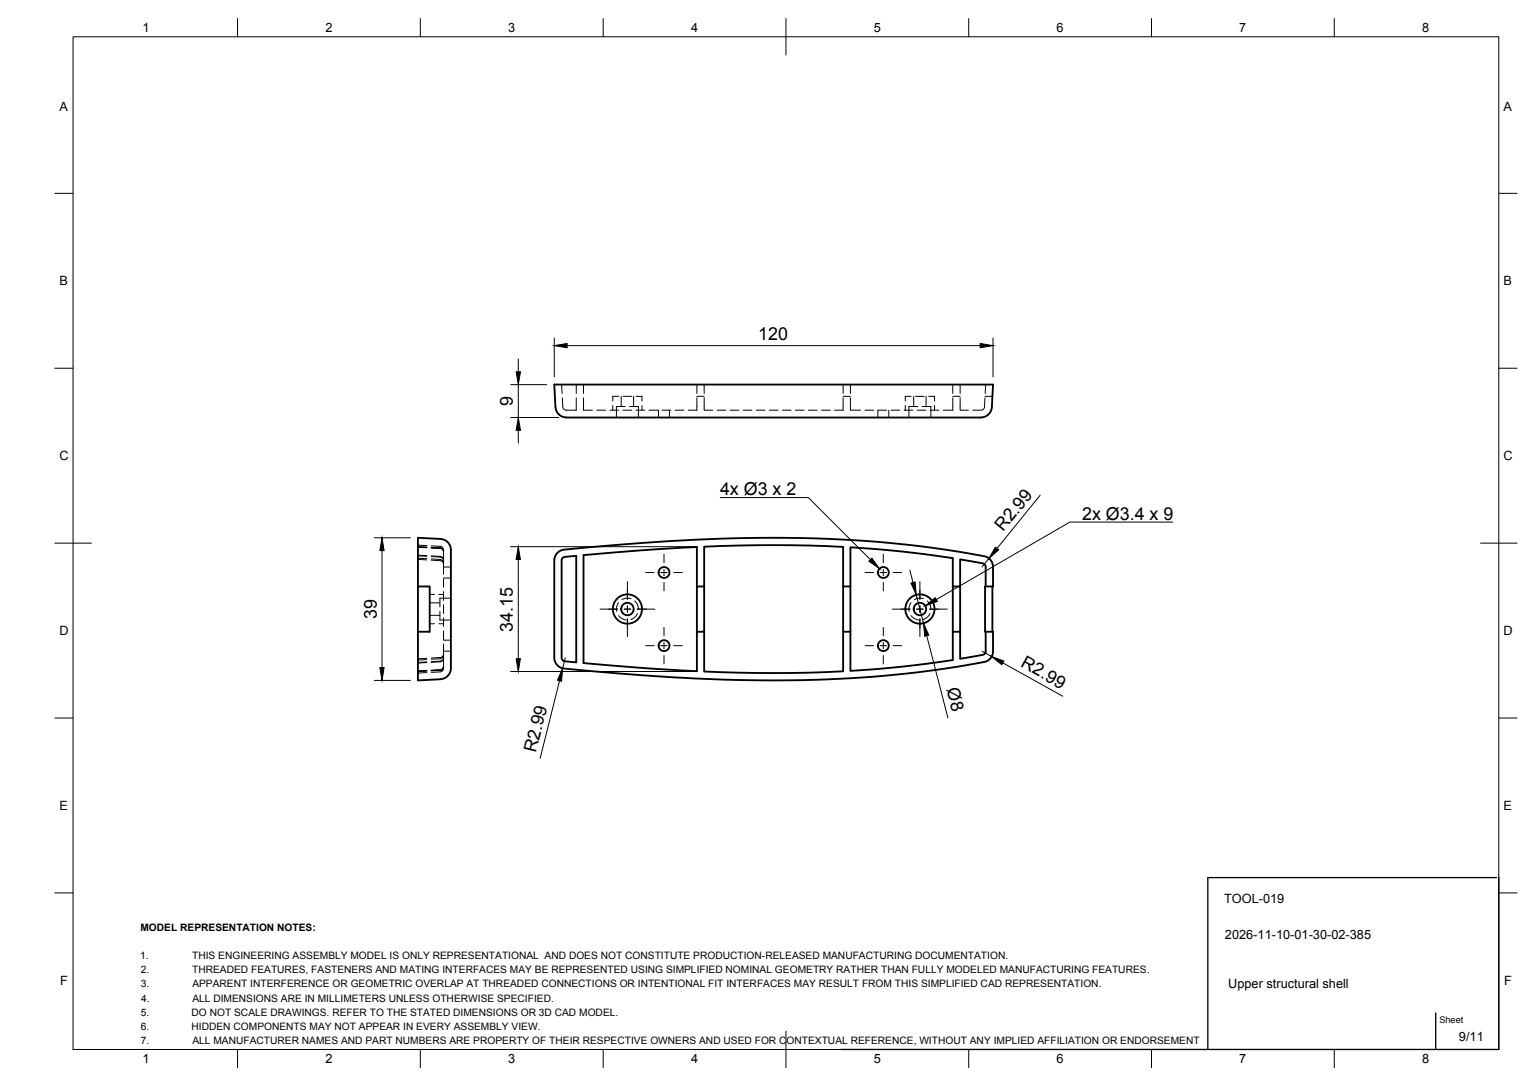
ISO-10303-21;
HEADER;
/* Generated by software containing ST-Developer
 * from STEP Tools, Inc. (www.steptools.com) 
 */

FILE_DESCRIPTION(
/* description */ (''),
/* implementation_level */ '2;1');

FILE_NAME(
/* name */ 'Upper structural shell.step',
/* time_stamp */ '2026-11-10T09:14:46-08:00',
/* author */ (''),
/* organization */ (''),
/* preprocessor_version */ 'ST-DEVELOPER v20.2',
/* originating_system */ 'Autodesk Translation Framework v15.17.0.0',
/* authorisation */ '');

FILE_SCHEMA (('AUTOMOTIVE_DESIGN { 1 0 10303 214 3 1 1 }'));
ENDSEC;

DATA;
#10=MECHANICAL_DESIGN_GEOMETRIC_PRESENTATION_REPRESENTATION('',(#562),#19471);
#76=SPHERICAL_SURFACE('',#7488,0.0999999999999999);
#77=SPHERICAL_SURFACE('',#7491,0.100000000000002);
#78=SPHERICAL_SURFACE('',#7495,0.0999999999999991);
#79=SPHERICAL_SURFACE('',#7499,0.1);
#80=SPHERICAL_SURFACE('',#7504,0.3);
#81=SPHERICAL_SURFACE('',#7508,0.300000000000002);
#82=SPHERICAL_SURFACE('',#7512,0.299999999999999);
#83=SPHERICAL_SURFACE('',#7517,0.3);
#92=B_SPLINE_SURFACE_WITH_KNOTS('',3,3,((#10686,#10687,#10688,#10689),(#10690,
#10691,#10692,#10693),(#10694,#10695,#10696,#10697),(#10698,#10699,#10700,
#10701)),.UNSPECIFIED.,.F.,.F.,.F.,(4,4),(4,4),(0.0627625298587661,0.3242096015809),
(0.0118073085896899,0.685451490706028),.UNSPECIFIED.);
#93=B_SPLINE_SURFACE_WITH_KNOTS('',3,3,((#10706,#10707,#10708,#10709),(#10710,
#10711,#10712,#10713),(#10714,#10715,#10716,#10717),(#10718,#10719,#10720,
#10721)),.UNSPECIFIED.,.F.,.F.,.F.,(4,4),(4,4),(0.0225360950145449,0.0483865590996774),
(0.0125659096559557,0.685650832343257),.UNSPECIFIED.);
#94=B_SPLINE_SURFACE_WITH_KNOTS('',3,3,((#10731,#10732,#10733,#10734),(#10735,
#10736,#10737,#10738),(#10739,#10740,#10741,#10742),(#10743,#10744,#10745,
#10746),(#10747,#10748,#10749,#10750)),.UNSPECIFIED.,.F.,.F.,.F.,(4,1,4),
(4,4),(0.,0.571428571428571,1.),(0.74118252158834,3.85438678954986),
 .UNSPECIFIED.);
#95=B_SPLINE_SURFACE_WITH_KNOTS('',3,3,((#10755,#10756,#10757,#10758),(#10759,
#10760,#10761,#10762),(#10763,#10764,#10765,#10766),(#10767,#10768,#10769,
#10770),(#10771,#10772,#10773,#10774)),.UNSPECIFIED.,.F.,.F.,.F.,(4,1,4),
(4,4),(0.,0.571428571428571,1.),(0.270878787657975,0.54981857912664),
 .UNSPECIFIED.);
#96=B_SPLINE_SURFACE_WITH_KNOTS('',3,3,((#10793,#10794,#10795,#10796),(#10797,
#10798,#10799,#10800),(#10801,#10802,#10803,#10804),(#10805,#10806,#10807,
#10808),(#10809,#10810,#10811,#10812)),.UNSPECIFIED.,.F.,.F.,.F.,(4,1,4),
(4,4),(0.,0.571428571428571,1.),(8.03948512627517,11.1526893942367),
 .UNSPECIFIED.);
#97=B_SPLINE_SURFACE_WITH_KNOTS('',3,3,((#10817,#10818,#10819,#10820),(#10821,
#10822,#10823,#10824),(#10825,#10826,#10827,#10828),(#10829,#10830,#10831,
#10832)),.UNSPECIFIED.,.F.,.F.,.F.,(4,4),(4,4),(0.675790398419059,0.937237470141233),
(0.0118073085603101,0.685451490706029),.UNSPECIFIED.);
#98=B_SPLINE_SURFACE_WITH_KNOTS('',3,3,((#10833,#10834,#10835,#10836),(#10837,
#10838,#10839,#10840),(#10841,#10842,#10843,#10844),(#10845,#10846,#10847,
#10848)),.UNSPECIFIED.,.F.,.F.,.F.,(4,4),(4,4),(0.951613440900322,0.977463904985455),
(0.0125659096559558,0.685650832343257),.UNSPECIFIED.);
#99=B_SPLINE_SURFACE_WITH_KNOTS('',3,3,((#10932,#10933,#10934,#10935),(#10936,
#10937,#10938,#10939),(#10940,#10941,#10942,#10943),(#10944,#10945,#10946,
#10947)),.UNSPECIFIED.,.F.,.F.,.F.,(4,4),(4,4),(0.340089900275858,0.660082688299826),
(0.0116294244283504,0.684384408933581),.UNSPECIFIED.);
#100=B_SPLINE_SURFACE_WITH_KNOTS('',3,3,((#10952,#10953,#10954,#10955),
(#10956,#10957,#10958,#10959),(#10960,#10961,#10962,#10963),(#10964,#10965,
#10966,#10967),(#10968,#10969,#10970,#10971)),.UNSPECIFIED.,.F.,.F.,.F.,
(4,1,4),(4,4),(0.,0.571428571428571,1.),(4.04989375377528,7.85140214144331),
 .UNSPECIFIED.);
#101=B_SPLINE_SURFACE_WITH_KNOTS('',3,3,((#10981,#10982,#10983,#10984),
(#10985,#10986,#10987,#10988),(#10989,#10990,#10991,#10992),(#10993,#10994,
#10995,#10996),(#10997,#10998,#10999,#11000)),.UNSPECIFIED.,.F.,.F.,.F.,
(4,1,4),(4,4),(0.,0.571428571428571,1.),(4.0424697743818,7.84397816204974),
 .UNSPECIFIED.);
#102=B_SPLINE_SURFACE_WITH_KNOTS('',3,3,((#11005,#11006,#11007,#11008),
(#11009,#11010,#11011,#11012),(#11013,#11014,#11015,#11016),(#11017,#11018,
#11019,#11020)),.UNSPECIFIED.,.F.,.F.,.F.,(4,4),(4,4),(0.339917311700174,
0.659910099724142),(0.0116294573698948,0.684384408933581),.UNSPECIFIED.);
#103=B_SPLINE_SURFACE_WITH_KNOTS('',3,3,((#11095,#11096,#11097,#11098),
(#11099,#11100,#11101,#11102),(#11103,#11104,#11105,#11106),(#11107,#11108,
#11109,#11110)),.UNSPECIFIED.,.F.,.F.,.F.,(4,4),(4,4),(0.675996615945502,
0.913173856075534),(0.0118505108223707,0.686152089762332),.UNSPECIFIED.);
#104=B_SPLINE_SURFACE_WITH_KNOTS('',3,3,((#11115,#11116,#11117,#11118),
(#11119,#11120,#11121,#11122),(#11123,#11124,#11125,#11126),(#11127,#11128,
#11129,#11130),(#11131,#11132,#11133,#11134)),.UNSPECIFIED.,.F.,.F.,.F.,
(4,1,4),(4,4),(0.,0.571428571428571,1.),(8.0457708503995,10.8690635835914),
 .UNSPECIFIED.);
#105=B_SPLINE_SURFACE_WITH_KNOTS('',3,3,((#11144,#11145,#11146,#11147),
(#11148,#11149,#11150,#11151),(#11152,#11153,#11154,#11155),(#11156,#11157,
#11158,#11159),(#11160,#11161,#11162,#11163)),.UNSPECIFIED.,.F.,.F.,.F.,
(4,1,4),(4,4),(0.,0.571428571428571,1.),(1.02480833223363,3.8481010654256),
 .UNSPECIFIED.);
#106=B_SPLINE_SURFACE_WITH_KNOTS('',3,3,((#11168,#11169,#11170,#11171),
(#11172,#11173,#11174,#11175),(#11176,#11177,#11178,#11179),(#11180,#11181,
#11182,#11183)),.UNSPECIFIED.,.F.,.F.,.F.,(4,4),(4,4),(0.0868261439244655,
0.324003384054498),(0.0118505108223707,0.686152089762332),.UNSPECIFIED.);
#107=B_SPLINE_SURFACE_WITH_KNOTS('',3,3,((#11258,#11259,#11260,#11261),
(#11262,#11263,#11264,#11265),(#11266,#11267,#11268,#11269),(#11270,#11271,
#11272,#11273)),.UNSPECIFIED.,.F.,.F.,.F.,(4,4),(4,4),(0.927751606342899,
0.979699913047832),(0.0130895688562318,0.686930956013783),.UNSPECIFIED.);
#108=B_SPLINE_SURFACE_WITH_KNOTS('',3,3,((#11283,#11284,#11285,#11286),
(#11287,#11288,#11289,#11290),(#11291,#11292,#11293,#11294),(#11295,#11296,
#11297,#11298),(#11299,#11300,#11301,#11302)),.UNSPECIFIED.,.F.,.F.,.F.,
(4,1,4),(4,4),(0.,0.571428571428571,1.),(11.0550486447215,11.6488871259622),
 .UNSPECIFIED.);
#109=B_SPLINE_SURFACE_WITH_KNOTS('',3,3,((#11316,#11317,#11318,#11319),
(#11320,#11321,#11322,#11323),(#11324,#11325,#11326,#11327),(#11328,#11329,
#11330,#11331)),.UNSPECIFIED.,.F.,.F.,.F.,(4,4),(4,4),(0.0203000869521683,
0.0722483936571013),(0.0130895688562318,0.686930956013783),
 .UNSPECIFIED.);
#110=B_SPLINE_SURFACE_WITH_KNOTS('',3,3,((#11341,#11342,#11343,#11344),
(#11345,#11346,#11347,#11348),(#11349,#11350,#11351,#11352),(#11353,#11354,
#11355,#11356),(#11357,#11358,#11359,#11360)),.UNSPECIFIED.,.F.,.F.,.F.,
(4,1,4),(4,4),(0.,0.571428571428571,1.),(0.244984789862841,0.838823271103535),
 .UNSPECIFIED.);
#111=B_SPLINE_SURFACE_WITH_KNOTS('',3,3,((#11374,#11375,#11376,#11377),
(#11378,#11379,#11380,#11381),(#11382,#11383,#11384,#11385),(#11386,#11387,
#11388,#11389),(#11390,#11391,#11392,#11393)),.UNSPECIFIED.,.F.,.F.,.F.,
(4,1,4),(4,4),(0.,0.5,1.),(0.0108921325678979,0.619909717328002),
 .UNSPECIFIED.);
#112=B_SPLINE_SURFACE_WITH_KNOTS('',3,3,((#11400,#11401,#11402,#11403),
(#11404,#11405,#11406,#11407),(#11408,#11409,#11410,#11411),(#11412,#11413,
#11414,#11415),(#11416,#11417,#11418,#11419)),.UNSPECIFIED.,.F.,.F.,.F.,
(4,1,4),(4,4),(0.,0.571428571428571,1.),(0.00967450486392679,0.618764321025346),
 .UNSPECIFIED.);
#113=B_SPLINE_SURFACE_WITH_KNOTS('',3,3,((#11424,#11425,#11426,#11427),
(#11428,#11429,#11430,#11431),(#11432,#11433,#11434,#11435),(#11436,#11437,
#11438,#11439),(#11440,#11441,#11442,#11443)),.UNSPECIFIED.,.F.,.F.,.F.,
(4,1,4),(4,4),(0.,0.571428571428571,1.),(0.0097274579809394,0.618764321025346),
 .UNSPECIFIED.);
#114=B_SPLINE_SURFACE_WITH_KNOTS('',3,3,((#11448,#11449,#11450,#11451),
(#11452,#11453,#11454,#11455),(#11456,#11457,#11458,#11459),(#11460,#11461,
#11462,#11463),(#11464,#11465,#11466,#11467)),.UNSPECIFIED.,.F.,.F.,.F.,
(4,1,4),(4,4),(0.,0.571428571428571,1.),(11.3440533366984,11.6229931281671),
 .UNSPECIFIED.);
#115=B_SPLINE_SURFACE_WITH_KNOTS('',3,3,((#11468,#11469,#11470,#11471),
(#11472,#11473,#11474,#11475),(#11476,#11477,#11478,#11479),(#11480,#11481,
#11482,#11483),(#11484,#11485,#11486,#11487)),.UNSPECIFIED.,.F.,.F.,.F.,
(4,1,4),(4,4),(0.,0.5,1.),(0.0108402259132964,0.619909717328002),
 .UNSPECIFIED.);
#116=B_SPLINE_SURFACE_WITH_KNOTS('',3,3,((#11513,#11514,#11515,#11516),
(#11517,#11518,#11519,#11520),(#11521,#11522,#11523,#11524),(#11525,#11526,
#11527,#11528),(#11529,#11530,#11531,#11532)),.UNSPECIFIED.,.F.,.F.,.F.,
(4,1,4),(4,4),(0.,0.571428571428571,1.),(-0.00387706229521417,0.619909717328002),
 .UNSPECIFIED.);
#117=B_SPLINE_SURFACE_WITH_KNOTS('',3,3,((#11551,#11552,#11553,#11554,#11555,
#11556),(#11557,#11558,#11559,#11560,#11561,#11562),(#11563,#11564,#11565,
#11566,#11567,#11568),(#11569,#11570,#11571,#11572,#11573,#11574),(#11575,
#11576,#11577,#11578,#11579,#11580)),.UNSPECIFIED.,.F.,.F.,.F.,(4,1,4),
(4,1,1,4),(0.,0.571428571428571,1.),(0.270878787657975,5.14716807550265,
8.39802760073243,11.6488871259622),.UNSPECIFIED.);
#118=B_SPLINE_SURFACE_WITH_KNOTS('',3,3,((#11593,#11594,#11595,#11596),
(#11597,#11598,#11599,#11600),(#11601,#11602,#11603,#11604),(#11605,#11606,
#11607,#11608),(#11609,#11610,#11611,#11612)),.UNSPECIFIED.,.F.,.F.,.F.,
(4,1,4),(4,4),(0.,0.571428571428571,1.),(-0.00522825793187074,0.618764321025346),
 .UNSPECIFIED.);
#119=B_SPLINE_SURFACE_WITH_KNOTS('',3,3,((#11621,#11622,#11623,#11624),
(#11625,#11626,#11627,#11628),(#11629,#11630,#11631,#11632),(#11633,#11634,
#11635,#11636),(#11637,#11638,#11639,#11640)),.UNSPECIFIED.,.F.,.F.,.F.,
(4,1,4),(4,4),(0.,0.571428571428571,1.),(-0.00506942997988007,0.618764321025346),
 .UNSPECIFIED.);
#120=B_SPLINE_SURFACE_WITH_KNOTS('',3,3,((#11649,#11650,#11651,#11652,#11653),
(#11654,#11655,#11656,#11657,#11658),(#11659,#11660,#11661,#11662,#11663),
(#11664,#11665,#11666,#11667,#11668),(#11669,#11670,#11671,#11672,#11673)),
 .UNSPECIFIED.,.F.,.F.,.F.,(4,1,4),(4,1,4),(0.,0.571428571428571,1.),(0.244984789862841,
5.12127407770751,11.6229931281671),.UNSPECIFIED.);
#121=B_SPLINE_SURFACE_WITH_KNOTS('',3,3,((#11684,#11685,#11686,#11687),
(#11688,#11689,#11690,#11691),(#11692,#11693,#11694,#11695),(#11696,#11697,
#11698,#11699),(#11700,#11701,#11702,#11703)),.UNSPECIFIED.,.F.,.F.,.F.,
(4,1,4),(4,4),(0.,0.571428571428571,1.),(-0.00403278922781227,0.619909717328002),
 .UNSPECIFIED.);
#122=B_SPLINE_SURFACE_WITH_KNOTS('',3,3,((#11712,#11713,#11714,#11715),
(#11716,#11717,#11718,#11719),(#11720,#11721,#11722,#11723),(#11724,#11725,
#11726,#11727)),.UNSPECIFIED.,.F.,.F.,.F.,(4,4),(4,4),(0.0225340877622934,
0.979701609653785),(0.,0.686930956013783),.UNSPECIFIED.);
#123=B_SPLINE_SURFACE_WITH_KNOTS('',3,3,((#11730,#11731,#11732,#11733),
(#11734,#11735,#11736,#11737),(#11738,#11739,#11740,#11741),(#11742,#11743,
#11744,#11745)),.UNSPECIFIED.,.F.,.F.,.F.,(4,4),(4,4),(0.0202983903462145,
0.977465912237707),(0.,0.686930956013783),.UNSPECIFIED.);
#172=B_SPLINE_CURVE_WITH_KNOTS('',3,(#9958,#9959,#9960,#9961,#9962,#9963),
 .UNSPECIFIED.,.F.,.F.,(4,2,4),(-0.607240122656937,-0.303691721894415,-0.000634514333697656),
 .UNSPECIFIED.);
#173=B_SPLINE_CURVE_WITH_KNOTS('',3,(#9965,#9966,#9967,#9968,#9969,#9970,
#9971,#9972,#9973,#9974,#9975,#9976,#9977,#9978,#9979,#9980,#9981,#9982,
#9983,#9984,#9985,#9986,#9987,#9988,#9989,#9990,#9991,#9992),
 .UNSPECIFIED.,.F.,.F.,(4,3,3,3,3,3,3,3,3,4),(-0.152223584381152,-0.128403685910756,
-0.115058138924018,-0.0911105876986024,-0.0779275105489685,-0.0651650823668383,
-0.0413494676927402,-0.0389105926748606,-0.0151313403168948,0.),
 .UNSPECIFIED.);
#174=B_SPLINE_CURVE_WITH_KNOTS('',3,(#9996,#9997,#9998,#9999,#10000,#10001,
#10002,#10003,#10004,#10005,#10006,#10007,#10008,#10009,#10010,#10011,#10012,
#10013,#10014,#10015,#10016,#10017,#10018,#10019,#10020,#10021,#10022,#10023),
 .UNSPECIFIED.,.F.,.F.,(4,3,3,3,3,3,3,3,3,4),(-0.152249917238265,-0.128484865669312,
-0.115494642307313,-0.0916985948709881,-0.0870953287403626,-0.0787006597758974,
-0.0547717013112817,-0.0393956522318865,-0.0155460991587222,0.),
 .UNSPECIFIED.);
#175=B_SPLINE_CURVE_WITH_KNOTS('',3,(#10024,#10025,#10026,#10027,#10028,
#10029),.UNSPECIFIED.,.F.,.F.,(4,2,4),(-0.606785315485727,-0.30369188913634,
-0.000179692314978108),.UNSPECIFIED.);
#176=B_SPLINE_CURVE_WITH_KNOTS('',3,(#10034,#10035,#10036,#10037,#10038,
#10039),.UNSPECIFIED.,.F.,.F.,(4,2,4),(-0.606332812995025,-0.303737653350621,
-0.000161665236032726),.UNSPECIFIED.);
#177=B_SPLINE_CURVE_WITH_KNOTS('',3,(#10041,#10042,#10043,#10044,#10045,
#10046,#10047,#10048,#10049,#10050,#10051,#10052,#10053,#10054,#10055,#10056,
#10057,#10058,#10059,#10060,#10061,#10062,#10063,#10064,#10065,#10066,#10067,
#10068),.UNSPECIFIED.,.F.,.F.,(4,3,3,3,3,3,3,3,3,4),(-0.152301160038588,
-0.128555435257278,-0.115184785848022,-0.0912639339035621,-0.0780773216554274,
-0.065267350293706,-0.0414723266145325,-0.0390252168402571,-0.0152374671294611,
0.),.UNSPECIFIED.);
#178=B_SPLINE_CURVE_WITH_KNOTS('',3,(#10072,#10073,#10074,#10075,#10076,
#10077,#10078,#10079,#10080,#10081,#10082,#10083,#10084,#10085,#10086,#10087,
#10088,#10089,#10090,#10091,#10092,#10093,#10094,#10095,#10096,#10097,#10098,
#10099),.UNSPECIFIED.,.F.,.F.,(4,3,3,3,3,3,3,3,3,4),(-0.152307894271445,
-0.128535938708366,-0.115295945509717,-0.0915234088298753,-0.0870575315710991,
-0.0782740392368046,-0.0543664511067997,-0.0391484926712317,-0.0153774171089249,
0.),.UNSPECIFIED.);
#179=B_SPLINE_CURVE_WITH_KNOTS('',3,(#10101,#10102,#10103,#10104,#10105,
#10106),.UNSPECIFIED.,.F.,.F.,(4,2,4),(-0.607315067615316,-0.303737782617996,
-0.00114390098251854),.UNSPECIFIED.);
#180=B_SPLINE_CURVE_WITH_KNOTS('',3,(#10112,#10113,#10114,#10115,#10116,
#10117),.UNSPECIFIED.,.F.,.F.,(4,2,4),(-0.606335618682527,-0.303964064424246,
-0.000163142902895597),.UNSPECIFIED.);
#181=B_SPLINE_CURVE_WITH_KNOTS('',3,(#10119,#10120,#10121,#10122,#10123,
#10124,#10125,#10126,#10127,#10128,#10129,#10130,#10131,#10132,#10133,#10134,
#10135,#10136,#10137,#10138,#10139,#10140,#10141,#10142,#10143,#10144,#10145,
#10146),.UNSPECIFIED.,.F.,.F.,(4,3,3,3,3,3,3,3,3,4),(-0.152324888062519,
-0.128571266282871,-0.115187819092559,-0.0912644922975459,-0.0780623053857969,
-0.0652705430018984,-0.0414736125245103,-0.0390138150290758,-0.015226502089553,
0.),.UNSPECIFIED.);
#182=B_SPLINE_CURVE_WITH_KNOTS('',3,(#10150,#10151,#10152,#10153,#10154,
#10155,#10156,#10157,#10158,#10159,#10160,#10161,#10162,#10163,#10164,#10165,
#10166,#10167,#10168,#10169,#10170,#10171,#10172,#10173,#10174,#10175,#10176,
#10177),.UNSPECIFIED.,.F.,.F.,(4,3,3,3,3,3,3,3,3,4),(-0.152333600285603,
-0.128561769460285,-0.115331525958272,-0.0915566852459163,-0.0870792380259527,
-0.0783165909319309,-0.0544069520497563,-0.0391732033593778,-0.0153939862842036,
0.),.UNSPECIFIED.);
#183=B_SPLINE_CURVE_WITH_KNOTS('',3,(#10179,#10180,#10181,#10182,#10183,
#10184),.UNSPECIFIED.,.F.,.F.,(4,2,4),(-0.607765665607205,-0.303964210965506,
-0.00159316434717749),.UNSPECIFIED.);
#184=B_SPLINE_CURVE_WITH_KNOTS('',3,(#10190,#10191,#10192,#10193,#10194,
#10195),.UNSPECIFIED.,.F.,.F.,(4,2,4),(-0.608113833554089,-0.304405910662044,
-0.00120843896277512),.UNSPECIFIED.);
#185=B_SPLINE_CURVE_WITH_KNOTS('',3,(#10197,#10198,#10199,#10200,#10201,
#10202,#10203,#10204,#10205,#10206,#10207,#10208,#10209,#10210,#10211,#10212,
#10213,#10214,#10215,#10216,#10217,#10218,#10219,#10220,#10221,#10222,#10223,
#10224),.UNSPECIFIED.,.F.,.F.,(4,3,3,3,3,3,3,3,3,4),(-0.152638346832965,
-0.128647829044501,-0.117000727359648,-0.0929750760194364,-0.0775532335837778,
-0.065166230851578,-0.0413072760700971,-0.0386249916896363,-0.0148681833632798,
0.),.UNSPECIFIED.);
#186=B_SPLINE_CURVE_WITH_KNOTS('',3,(#10228,#10229,#10230,#10231,#10232,
#10233,#10234,#10235,#10236,#10237,#10238,#10239,#10240,#10241,#10242,#10243,
#10244,#10245,#10246,#10247,#10248,#10249,#10250,#10251,#10252,#10253,#10254,
#10255),.UNSPECIFIED.,.F.,.F.,(4,3,3,3,3,3,3,3,3,4),(-0.152712908768378,
-0.128963682254188,-0.116304008925778,-0.092453135123643,-0.0875380734791113,
-0.0797852913889514,-0.0558105568475602,-0.0400274901149945,-0.0159798645019078,
0.),.UNSPECIFIED.);
#187=B_SPLINE_CURVE_WITH_KNOTS('',3,(#10257,#10258,#10259,#10260,#10261,
#10262),.UNSPECIFIED.,.F.,.F.,(4,2,4),(-0.607607610897069,-0.304406883675693,
-0.000702187548907163),.UNSPECIFIED.);
#188=B_SPLINE_CURVE_WITH_KNOTS('',3,(#10268,#10269,#10270,#10271),
 .UNSPECIFIED.,.F.,.F.,(4,4),(0.0130288733793136,0.619909717328002),
 .UNSPECIFIED.);
#189=B_SPLINE_CURVE_WITH_KNOTS('',3,(#10275,#10276,#10277,#10278),
 .UNSPECIFIED.,.F.,.F.,(4,4),(-0.619909717328002,-0.0130288733793137),
 .UNSPECIFIED.);
#190=B_SPLINE_CURVE_WITH_KNOTS('',3,(#10281,#10282,#10283,#10284,#10285,
#10286,#10287),.UNSPECIFIED.,.F.,.F.,(4,3,4),(7.87274532319472,10.4298004347969,
10.9780233963721),.UNSPECIFIED.);
#191=B_SPLINE_CURVE_WITH_KNOTS('',3,(#10288,#10289,#10290,#10291,#10292,
#10293,#10294),.UNSPECIFIED.,.F.,.F.,(4,3,4),(0.511752108249611,2.84807862798167,
3.61537599721027),.UNSPECIFIED.);
#192=B_SPLINE_CURVE_WITH_KNOTS('',3,(#10297,#10298,#10299,#10300,#10301,
#10302,#10303),.UNSPECIFIED.,.F.,.F.,(4,3,4),(3.81523717927831,5.72635044542746,
7.61820606472736),.UNSPECIFIED.);
#193=B_SPLINE_CURVE_WITH_KNOTS('',3,(#10306,#10307,#10308,#10309),
 .UNSPECIFIED.,.F.,.F.,(4,4),(7.8195516254834,10.6519234170402),
 .UNSPECIFIED.);
#194=B_SPLINE_CURVE_WITH_KNOTS('',3,(#10313,#10314,#10315,#10316),
 .UNSPECIFIED.,.F.,.F.,(4,4),(10.8550709503701,11.4839159448819),
 .UNSPECIFIED.);
#195=B_SPLINE_CURVE_WITH_KNOTS('',3,(#10317,#10318,#10319,#10320,#10321,
#10322,#10323,#10324,#10325,#10326,#10327,#10328,#10329,#10330,#10331,#10332,
#10333,#10334,#10335,#10336,#10337,#10338,#10339,#10340,#10341,#10342,#10343,
#10344),.UNSPECIFIED.,.F.,.F.,(4,3,3,3,3,3,3,3,3,4),(0.,0.023800266251022,
0.0390470051780055,0.062864594207143,0.0692752090304052,0.0780196763370091,
0.101808338076191,0.108235461704482,0.131970324379069,0.138468980573541),
 .UNSPECIFIED.);
#196=B_SPLINE_CURVE_WITH_KNOTS('',3,(#10348,#10349,#10350,#10351,#10352,
#10353,#10354,#10355,#10356,#10357,#10358,#10359,#10360,#10361,#10362,#10363,
#10364,#10365,#10366,#10367,#10368,#10369,#10370,#10371,#10372,#10373,#10374,
#10375,#10376,#10377,#10378),.UNSPECIFIED.,.F.,.F.,(4,3,3,3,3,3,3,3,3,3,
4),(0.,0.0536158767337707,0.107707970980176,0.117140678528723,0.171373940961503,
0.178118425384842,0.234058785038521,0.2884659822146,0.324708667187819,0.378759781373182,
0.415412568437851),.UNSPECIFIED.);
#197=B_SPLINE_CURVE_WITH_KNOTS('',3,(#10380,#10381,#10382,#10383),
 .UNSPECIFIED.,.F.,.F.,(4,4),(0.0202983903462145,0.977465912237707),
 .UNSPECIFIED.);
#198=B_SPLINE_CURVE_WITH_KNOTS('',3,(#10385,#10386,#10387,#10388,#10389,
#10390,#10391,#10392,#10393,#10394,#10395,#10396,#10397,#10398,#10399,#10400,
#10401,#10402,#10403,#10404,#10405,#10406,#10407,#10408,#10409,#10410,#10411,
#10412,#10413,#10414,#10415),.UNSPECIFIED.,.F.,.F.,(4,3,3,3,3,3,3,3,3,3,
4),(0.,0.053547205187505,0.107728964525782,0.117299670245694,0.171524652009909,
0.189842726242433,0.234296321023441,0.288773621215207,0.338477936388461,
0.392564001789548,0.442713223041249),.UNSPECIFIED.);
#199=B_SPLINE_CURVE_WITH_KNOTS('',3,(#10419,#10420,#10421,#10422,#10423,
#10424,#10425,#10426,#10427,#10428,#10429,#10430,#10431,#10432,#10433,#10434,
#10435,#10436,#10437,#10438,#10439,#10440,#10441,#10442,#10443,#10444,#10445,
#10446,#10447,#10448,#10449),.UNSPECIFIED.,.F.,.F.,(4,3,3,3,3,3,3,3,3,3,
4),(0.,0.0535312152416108,0.107707123412492,0.117215931328448,0.171445047002381,
0.189808362521926,0.234165405003858,0.288639615809812,0.338404447092272,
0.392504428396833,0.442708851597914),.UNSPECIFIED.);
#200=B_SPLINE_CURVE_WITH_KNOTS('',3,(#10451,#10452,#10453,#10454),
 .UNSPECIFIED.,.F.,.F.,(4,4),(0.0225340877622936,0.979701609653785),
 .UNSPECIFIED.);
#201=B_SPLINE_CURVE_WITH_KNOTS('',3,(#10456,#10457,#10458,#10459,#10460,
#10461,#10462,#10463,#10464,#10465,#10466,#10467,#10468,#10469,#10470,#10471,
#10472,#10473,#10474,#10475,#10476,#10477,#10478,#10479,#10480,#10481,#10482,
#10483,#10484,#10485,#10486),.UNSPECIFIED.,.F.,.F.,(4,3,3,3,3,3,3,3,3,3,
4),(0.,0.0536458552170769,0.107744721567334,0.117297895480617,0.171522683869793,
0.178177673384308,0.23429412186666,0.288702228477357,0.324838815929715,
0.378862861687027,0.415420074045746),.UNSPECIFIED.);
#202=B_SPLINE_CURVE_WITH_KNOTS('',3,(#10489,#10490,#10491,#10492,#10493,
#10494,#10495,#10496,#10497,#10498,#10499,#10500,#10501,#10502,#10503,#10504,
#10505,#10506,#10507,#10508,#10509,#10510,#10511,#10512,#10513,#10514,#10515,
#10516),.UNSPECIFIED.,.F.,.F.,(4,3,3,3,3,3,3,3,3,4),(0.,0.0238098951475563,
0.0390995920428052,0.0629117710415135,0.0692953339558167,0.0780985718814299,
0.101889748471939,0.108278926258091,0.132003149848588,0.138471484390145),
 .UNSPECIFIED.);
#203=B_SPLINE_CURVE_WITH_KNOTS('',3,(#10518,#10519,#10520,#10521),
 .UNSPECIFIED.,.F.,.F.,(4,4),(2.05597917304345E-5,0.629200412657851),
 .UNSPECIFIED.);
#204=B_SPLINE_CURVE_WITH_KNOTS('',3,(#10524,#10525,#10526,#10527),
 .UNSPECIFIED.,.F.,.F.,(4,4),(0.832456091119126,3.6663340257767),
 .UNSPECIFIED.);
#205=B_SPLINE_CURVE_WITH_KNOTS('',3,(#10530,#10531,#10532,#10533,#10534,
#10535,#10536),.UNSPECIFIED.,.F.,.F.,(4,3,4),(3.86778652923942,5.76006783397632,
7.67277763234621),.UNSPECIFIED.);
#206=B_SPLINE_CURVE_WITH_KNOTS('',3,(#10540,#10541,#10542,#10543),
 .UNSPECIFIED.,.F.,.F.,(4,4),(11.1789026308149,11.490024089745),
 .UNSPECIFIED.);
#207=B_SPLINE_CURVE_WITH_KNOTS('',3,(#10545,#10546,#10547,#10548,#10549,
#10550,#10551,#10552,#10553,#10554,#10555,#10556,#10557,#10558,#10559,#10560,
#10561,#10562,#10563,#10564,#10565,#10566,#10567,#10568,#10569),
 .UNSPECIFIED.,.F.,.F.,(4,3,3,3,3,3,3,3,4),(0.,0.0238050540413609,0.0390723036702896,
0.0632692088215501,0.0780555758269344,0.101951849921082,0.112801451778717,
0.136536488207902,0.147568670144067),.UNSPECIFIED.);
#208=B_SPLINE_CURVE_WITH_KNOTS('',3,(#10573,#10574,#10575,#10576,#10577,
#10578,#10579,#10580,#10581,#10582,#10583,#10584,#10585,#10586,#10587,#10588,
#10589,#10590,#10591,#10592,#10593,#10594,#10595,#10596,#10597),
 .UNSPECIFIED.,.F.,.F.,(4,3,3,3,3,3,3,3,4),(0.,0.0238098889950854,0.0391003179068551,
0.0632803937136523,0.0780994777107358,0.101997157448698,0.112825962756833,
0.136555142506291,0.147570127973408),.UNSPECIFIED.);
#209=B_SPLINE_CURVE_WITH_KNOTS('',3,(#10599,#10600,#10601,#10602),
 .UNSPECIFIED.,.F.,.F.,(4,4),(2.41556456535008E-5,0.310979882704647),
 .UNSPECIFIED.);
#210=B_SPLINE_CURVE_WITH_KNOTS('',3,(#10614,#10615,#10616,#10617,#10618,
#10619),.UNSPECIFIED.,.F.,.F.,(4,2,4),(-0.606744425054929,-0.30369469419025,
-0.000104868936493974),.UNSPECIFIED.);
#211=B_SPLINE_CURVE_WITH_KNOTS('',3,(#10621,#10622,#10623,#10624,#10625,
#10626),.UNSPECIFIED.,.F.,.F.,(4,2,4),(-0.60732337425873,-0.303694522808999,
-0.000683832228057069),.UNSPECIFIED.);
#212=B_SPLINE_CURVE_WITH_KNOTS('',3,(#10628,#10629,#10630,#10631,#10632,
#10633,#10634,#10635,#10636,#10637,#10638,#10639,#10640,#10641,#10642,#10643,
#10644,#10645,#10646,#10647,#10648,#10649,#10650,#10651,#10652,#10653,#10654,
#10655),.UNSPECIFIED.,.F.,.F.,(4,3,3,3,3,3,3,3,3,4),(-0.152213081758773,
-0.128388856548194,-0.115047734630008,-0.0910986092737131,-0.0779187269986961,
-0.0651565114518209,-0.0413397067626705,-0.0389038209724845,-0.0151251319644201,
0.),.UNSPECIFIED.);
#213=B_SPLINE_CURVE_WITH_KNOTS('',3,(#10658,#10659,#10660,#10661,#10662,
#10663,#10664,#10665,#10666,#10667,#10668,#10669,#10670,#10671,#10672,#10673,
#10674,#10675,#10676,#10677,#10678,#10679,#10680,#10681,#10682,#10683,#10684,
#10685),.UNSPECIFIED.,.F.,.F.,(4,3,3,3,3,3,3,3,3,4),(-0.152240567100014,
-0.128476012965191,-0.115503482174674,-0.0917060839439778,-0.0870941983819305,
-0.0787260045726768,-0.0547958477503903,-0.0394103419198022,-0.0155561788900784,
0.),.UNSPECIFIED.);
#214=B_SPLINE_CURVE_WITH_KNOTS('',3,(#10702,#10703,#10704,#10705),
 .UNSPECIFIED.,.F.,.F.,(4,4),(-3.85438678954986,-0.750511952447855),
 .UNSPECIFIED.);
#215=B_SPLINE_CURVE_WITH_KNOTS('',3,(#10723,#10724,#10725,#10726),
 .UNSPECIFIED.,.F.,.F.,(4,4),(-0.54981857912664,-0.270878787657975),
 .UNSPECIFIED.);
#216=B_SPLINE_CURVE_WITH_KNOTS('',3,(#10727,#10728,#10729,#10730),
 .UNSPECIFIED.,.F.,.F.,(4,4),(-0.618764321025346,-0.0114172178585034),
 .UNSPECIFIED.);
#217=B_SPLINE_CURVE_WITH_KNOTS('',3,(#10751,#10752,#10753,#10754),
 .UNSPECIFIED.,.F.,.F.,(4,4),(0.74118252158834,3.84969085360113),
 .UNSPECIFIED.);
#218=B_SPLINE_CURVE_WITH_KNOTS('',3,(#10776,#10777,#10778,#10779),
 .UNSPECIFIED.,.F.,.F.,(4,4),(0.270878787657975,0.540284107299618),
 .UNSPECIFIED.);
#219=B_SPLINE_CURVE_WITH_KNOTS('',3,(#10782,#10783,#10784,#10785),
 .UNSPECIFIED.,.F.,.F.,(4,4),(8.04418106222393,11.1526893942367),
 .UNSPECIFIED.);
#220=B_SPLINE_CURVE_WITH_KNOTS('',3,(#10788,#10789,#10790,#10791),
 .UNSPECIFIED.,.F.,.F.,(4,4),(11.3535878085254,11.6229931281671),
 .UNSPECIFIED.);
#221=B_SPLINE_CURVE_WITH_KNOTS('',3,(#10813,#10814,#10815,#10816),
 .UNSPECIFIED.,.F.,.F.,(4,4),(-11.1433599633772,-8.03948512627517),
 .UNSPECIFIED.);
#222=B_SPLINE_CURVE_WITH_KNOTS('',3,(#10850,#10851,#10852,#10853),
 .UNSPECIFIED.,.F.,.F.,(4,4),(0.0114172178585033,0.618764321025346),
 .UNSPECIFIED.);
#223=B_SPLINE_CURVE_WITH_KNOTS('',3,(#10854,#10855,#10856,#10857),
 .UNSPECIFIED.,.F.,.F.,(4,4),(-11.6229931281671,-11.3440533366984),
 .UNSPECIFIED.);
#224=B_SPLINE_CURVE_WITH_KNOTS('',3,(#10860,#10861,#10862,#10863,#10864,
#10865),.UNSPECIFIED.,.F.,.F.,(4,2,4),(-0.606286853269513,-0.303735636734938,
-0.000134370544016882),.UNSPECIFIED.);
#225=B_SPLINE_CURVE_WITH_KNOTS('',3,(#10867,#10868,#10869,#10870,#10871,
#10872,#10873,#10874,#10875,#10876,#10877,#10878,#10879,#10880,#10881,#10882,
#10883,#10884,#10885,#10886,#10887,#10888,#10889,#10890,#10891,#10892,#10893,
#10894),.UNSPECIFIED.,.F.,.F.,(4,3,3,3,3,3,3,3,3,4),(-0.152301724526365,
-0.128559761662057,-0.115189905045126,-0.0912708316251271,-0.0780855696141105,
-0.0652713768517459,-0.0414777101816728,-0.0390314967756457,-0.015242903619151,
0.),.UNSPECIFIED.);
#226=B_SPLINE_CURVE_WITH_KNOTS('',3,(#10898,#10899,#10900,#10901,#10902,
#10903,#10904,#10905,#10906,#10907,#10908,#10909,#10910,#10911,#10912,#10913,
#10914,#10915,#10916,#10917,#10918,#10919,#10920,#10921,#10922,#10923,#10924,
#10925),.UNSPECIFIED.,.F.,.F.,(4,3,3,3,3,3,3,3,3,4),(-0.1523073815286,-0.1285346644938,
-0.115283264026726,-0.0915123087981378,-0.0870533687950649,-0.0782507800682277,
-0.0543447803816484,-0.0391350231834537,-0.0153679399182895,0.),
 .UNSPECIFIED.);
#227=B_SPLINE_CURVE_WITH_KNOTS('',3,(#10926,#10927,#10928,#10929,#10930,
#10931),.UNSPECIFIED.,.F.,.F.,(4,2,4),(-0.607338074051965,-0.303735662161239,
-0.00118557149519966),.UNSPECIFIED.);
#228=B_SPLINE_CURVE_WITH_KNOTS('',3,(#10948,#10949,#10950,#10951),
 .UNSPECIFIED.,.F.,.F.,(4,4),(-7.8460657686783,-4.05419673417835),
 .UNSPECIFIED.);
#229=B_SPLINE_CURVE_WITH_KNOTS('',3,(#10972,#10973,#10974,#10975),
 .UNSPECIFIED.,.F.,.F.,(4,4),(4.04989375377528,7.85140214144331),
 .UNSPECIFIED.);
#230=B_SPLINE_CURVE_WITH_KNOTS('',3,(#10977,#10978,#10979,#10980),
 .UNSPECIFIED.,.F.,.F.,(4,4),(4.0424697743818,7.84397816204974),
 .UNSPECIFIED.);
#231=B_SPLINE_CURVE_WITH_KNOTS('',3,(#11001,#11002,#11003,#11004),
 .UNSPECIFIED.,.F.,.F.,(4,4),(-7.83967518164668,-4.0478061471468),
 .UNSPECIFIED.);
#232=B_SPLINE_CURVE_WITH_KNOTS('',3,(#11023,#11024,#11025,#11026,#11027,
#11028),.UNSPECIFIED.,.F.,.F.,(4,2,4),(-0.606398914035431,-0.303967092551845,
-0.000200694235479137),.UNSPECIFIED.);
#233=B_SPLINE_CURVE_WITH_KNOTS('',3,(#11030,#11031,#11032,#11033,#11034,
#11035,#11036,#11037,#11038,#11039,#11040,#11041,#11042,#11043,#11044,#11045,
#11046,#11047,#11048,#11049,#11050,#11051,#11052,#11053,#11054,#11055,#11056,
#11057),.UNSPECIFIED.,.F.,.F.,(4,3,3,3,3,3,3,3,3,4),(-0.15233244131821,
-0.128569871170003,-0.115181988990177,-0.0912564475476021,-0.0780459432968613,
-0.0652662335163151,-0.0414674738832469,-0.0390013640446512,-0.0152139229936509,
0.),.UNSPECIFIED.);
#234=B_SPLINE_CURVE_WITH_KNOTS('',3,(#11061,#11062,#11063,#11064,#11065,
#11066,#11067,#11068,#11069,#11070,#11071,#11072,#11073,#11074,#11075,#11076,
#11077,#11078,#11079,#11080,#11081,#11082,#11083,#11084,#11085,#11086,#11087,
#11088),.UNSPECIFIED.,.F.,.F.,(4,3,3,3,3,3,3,3,3,4),(-0.152343297533924,
-0.128571042154168,-0.115361098257144,-0.0915841820623439,-0.0870924557961151,
-0.0783628838319633,-0.0544516462338148,-0.0392000432438046,-0.0154115240971992,
0.),.UNSPECIFIED.);
#235=B_SPLINE_CURVE_WITH_KNOTS('',3,(#11089,#11090,#11091,#11092,#11093,
#11094),.UNSPECIFIED.,.F.,.F.,(4,2,4),(-0.607734321217702,-0.303967174049374,
-0.00153607519677973),.UNSPECIFIED.);
#236=B_SPLINE_CURVE_WITH_KNOTS('',3,(#11111,#11112,#11113,#11114),
 .UNSPECIFIED.,.F.,.F.,(4,4),(-10.8531956503852,-8.0457708503995),
 .UNSPECIFIED.);
#237=B_SPLINE_CURVE_WITH_KNOTS('',3,(#11135,#11136,#11137,#11138),
 .UNSPECIFIED.,.F.,.F.,(4,4),(8.05172912332209,10.8690635835914),
 .UNSPECIFIED.);
#238=B_SPLINE_CURVE_WITH_KNOTS('',3,(#11140,#11141,#11142,#11143),
 .UNSPECIFIED.,.F.,.F.,(4,4),(1.02480833223363,3.84214279250303),
 .UNSPECIFIED.);
#239=B_SPLINE_CURVE_WITH_KNOTS('',3,(#11164,#11165,#11166,#11167),
 .UNSPECIFIED.,.F.,.F.,(4,4),(-3.8481010654256,-1.04067626543981),
 .UNSPECIFIED.);
#240=B_SPLINE_CURVE_WITH_KNOTS('',3,(#11186,#11187,#11188,#11189,#11190,
#11191),.UNSPECIFIED.,.F.,.F.,(4,2,4),(-0.608301643694891,-0.304416323412316,
-0.0013178649037765),.UNSPECIFIED.);
#241=B_SPLINE_CURVE_WITH_KNOTS('',3,(#11193,#11194,#11195,#11196,#11197,
#11198,#11199,#11200,#11201,#11202,#11203,#11204,#11205,#11206,#11207,#11208,
#11209,#11210,#11211,#11212,#11213,#11214,#11215,#11216,#11217,#11218,#11219,
#11220),.UNSPECIFIED.,.F.,.F.,(4,3,3,3,3,3,3,3,3,4),(-0.152679905805259,
-0.128657903528546,-0.116982385578132,-0.0929502017086943,-0.0774957796939621,
-0.0651567901405441,-0.0412920018136918,-0.0385809476656748,-0.0148252868187304,
0.),.UNSPECIFIED.);
#242=B_SPLINE_CURVE_WITH_KNOTS('',3,(#11224,#11225,#11226,#11227,#11228,
#11229,#11230,#11231,#11232,#11233,#11234,#11235,#11236,#11237,#11238,#11239,
#11240,#11241,#11242,#11243,#11244,#11245,#11246,#11247,#11248,#11249,#11250,
#11251),.UNSPECIFIED.,.F.,.F.,(4,3,3,3,3,3,3,3,3,4),(-0.152762160496458,
-0.129013039804674,-0.116418683706179,-0.0925605502531877,-0.0875939536119484,
-0.0799546107253736,-0.055976748465099,-0.0401263304884301,-0.0160466564276224,
0.),.UNSPECIFIED.);
#243=B_SPLINE_CURVE_WITH_KNOTS('',3,(#11252,#11253,#11254,#11255,#11256,
#11257),.UNSPECIFIED.,.F.,.F.,(4,2,4),(-0.607519387555057,-0.304417308507995,
-0.000535579674449116),.UNSPECIFIED.);
#244=B_SPLINE_CURVE_WITH_KNOTS('',3,(#11275,#11276,#11277,#11278),
 .UNSPECIFIED.,.F.,.F.,(4,4),(0.012184405392802,0.619909717328002),
 .UNSPECIFIED.);
#245=B_SPLINE_CURVE_WITH_KNOTS('',3,(#11279,#11280,#11281,#11282),
 .UNSPECIFIED.,.F.,.F.,(4,4),(-11.6488871259622,-11.0550486447215),
 .UNSPECIFIED.);
#246=B_SPLINE_CURVE_WITH_KNOTS('',3,(#11305,#11306,#11307,#11308),
 .UNSPECIFIED.,.F.,.F.,(4,4),(11.0717103908866,11.6488871259622),
 .UNSPECIFIED.);
#247=B_SPLINE_CURVE_WITH_KNOTS('',3,(#11312,#11313,#11314,#11315),
 .UNSPECIFIED.,.F.,.F.,(4,4),(0.244984789862841,0.822161524938444),
 .UNSPECIFIED.);
#248=B_SPLINE_CURVE_WITH_KNOTS('',3,(#11333,#11334,#11335,#11336),
 .UNSPECIFIED.,.F.,.F.,(4,4),(-0.838823271103535,-0.244984789862841),
 .UNSPECIFIED.);
#249=B_SPLINE_CURVE_WITH_KNOTS('',3,(#11337,#11338,#11339,#11340),
 .UNSPECIFIED.,.F.,.F.,(4,4),(-0.619909717328002,-0.0121844053928019),
 .UNSPECIFIED.);
#250=B_SPLINE_CURVE_WITH_KNOTS('',3,(#11420,#11421,#11422,#11423),
 .UNSPECIFIED.,.F.,.F.,(4,4),(0.011877999214525,0.618764321025346),
 .UNSPECIFIED.);
#251=B_SPLINE_CURVE_WITH_KNOTS('',3,(#11444,#11445,#11446,#11447),
 .UNSPECIFIED.,.F.,.F.,(4,4),(-0.618764321025346,-0.0118779992145249),
 .UNSPECIFIED.);
#252=B_SPLINE_CURVE_WITH_KNOTS('',3,(#11533,#11534,#11535,#11536),
 .UNSPECIFIED.,.F.,.F.,(4,4),(-1.34441069388203E-17,0.619909717328002),
 .UNSPECIFIED.);
#253=B_SPLINE_CURVE_WITH_KNOTS('',3,(#11537,#11538,#11539,#11540),
 .UNSPECIFIED.,.F.,.F.,(4,4),(-0.619909717328002,-0.00253319281730041),
 .UNSPECIFIED.);
#254=B_SPLINE_CURVE_WITH_KNOTS('',3,(#11581,#11582,#11583,#11584,#11585,
#11586),.UNSPECIFIED.,.F.,.F.,(4,1,1,4),(-11.6488871259622,-8.39802760073243,
-5.14716807550265,-0.270878787657975),.UNSPECIFIED.);
#255=B_SPLINE_CURVE_WITH_KNOTS('',3,(#11587,#11588,#11589,#11590,#11591,
#11592),.UNSPECIFIED.,.F.,.F.,(4,1,1,4),(0.270878787657975,5.14716807550265,
8.39802760073243,11.6488871259622),.UNSPECIFIED.);
#256=B_SPLINE_CURVE_WITH_KNOTS('',3,(#11613,#11614,#11615,#11616),
 .UNSPECIFIED.,.F.,.F.,(4,4),(0.0013822243147816,0.618764321025346),
 .UNSPECIFIED.);
#257=B_SPLINE_CURVE_WITH_KNOTS('',3,(#11617,#11618,#11619,#11620),
 .UNSPECIFIED.,.F.,.F.,(4,4),(-0.618764321025346,8.06646416329215E-17),
 .UNSPECIFIED.);
#258=B_SPLINE_CURVE_WITH_KNOTS('',3,(#11641,#11642,#11643,#11644),
 .UNSPECIFIED.,.F.,.F.,(4,4),(-9.36750677027476E-17,0.618764321025346),
 .UNSPECIFIED.);
#259=B_SPLINE_CURVE_WITH_KNOTS('',3,(#11645,#11646,#11647,#11648),
 .UNSPECIFIED.,.F.,.F.,(4,4),(-0.618764321025346,-0.00138222431478148),
 .UNSPECIFIED.);
#260=B_SPLINE_CURVE_WITH_KNOTS('',3,(#11674,#11675,#11676,#11677,#11678),
 .UNSPECIFIED.,.F.,.F.,(4,1,4),(-11.6229931281671,-5.12127407770751,-0.244984789862841),
 .UNSPECIFIED.);
#261=B_SPLINE_CURVE_WITH_KNOTS('',3,(#11679,#11680,#11681,#11682,#11683),
 .UNSPECIFIED.,.F.,.F.,(4,1,4),(0.244984789862841,5.12127407770751,11.6229931281671),
 .UNSPECIFIED.);
#262=B_SPLINE_CURVE_WITH_KNOTS('',3,(#11704,#11705,#11706,#11707),
 .UNSPECIFIED.,.F.,.F.,(4,4),(0.00253319281730024,0.619909717328002),
 .UNSPECIFIED.);
#263=B_SPLINE_CURVE_WITH_KNOTS('',3,(#11708,#11709,#11710,#11711),
 .UNSPECIFIED.,.F.,.F.,(4,4),(-0.619909717328002,-2.51534904016637E-17),
 .UNSPECIFIED.);
#542=SHAPE_REPRESENTATION_RELATIONSHIP('SRR','None',#19522,#552);
#552=ADVANCED_BREP_SHAPE_REPRESENTATION('',(#572),#19465);
#562=STYLED_ITEM('',(#19584),#572);
#572=MANIFOLD_SOLID_BREP('Body1',#7155);
#601=FACE_BOUND('',#1337,.T.);
#602=FACE_BOUND('',#1340,.T.);
#603=FACE_BOUND('',#1351,.T.);
#604=FACE_BOUND('',#1353,.T.);
#605=FACE_BOUND('',#1365,.T.);
#606=FACE_BOUND('',#1374,.T.);
#607=FACE_BOUND('',#1375,.T.);
#608=FACE_BOUND('',#1376,.T.);
#609=FACE_BOUND('',#1391,.T.);
#610=FACE_BOUND('',#1392,.T.);
#611=FACE_BOUND('',#1393,.T.);
#612=FACE_BOUND('',#1429,.T.);
#613=FACE_BOUND('',#1430,.T.);
#614=FACE_BOUND('',#1431,.T.);
#615=FACE_BOUND('',#1432,.T.);
#616=FACE_BOUND('',#1433,.T.);
#617=FACE_BOUND('',#1434,.T.);
#706=PLANE('',#7439);
#707=PLANE('',#7444);
#708=PLANE('',#7450);
#709=PLANE('',#7451);
#710=PLANE('',#7452);
#711=PLANE('',#7453);
#712=PLANE('',#7454);
#713=PLANE('',#7455);
#714=PLANE('',#7456);
#715=PLANE('',#7457);
#716=PLANE('',#7459);
#717=PLANE('',#7461);
#718=PLANE('',#7462);
#719=PLANE('',#7463);
#720=PLANE('',#7464);
#721=PLANE('',#7465);
#722=PLANE('',#7466);
#723=PLANE('',#7467);
#724=PLANE('',#7468);
#725=PLANE('',#7469);
#726=PLANE('',#7470);
#727=PLANE('',#7471);
#728=PLANE('',#7476);
#729=PLANE('',#7478);
#730=PLANE('',#7479);
#731=PLANE('',#7480);
#732=PLANE('',#7481);
#733=PLANE('',#7482);
#734=PLANE('',#7483);
#735=PLANE('',#7484);
#736=PLANE('',#7486);
#737=PLANE('',#7503);
#738=PLANE('',#7522);
#739=PLANE('',#7523);
#740=PLANE('',#7524);
#903=FACE_OUTER_BOUND('',#1331,.T.);
#904=FACE_OUTER_BOUND('',#1332,.T.);
#905=FACE_OUTER_BOUND('',#1333,.T.);
#906=FACE_OUTER_BOUND('',#1334,.T.);
#907=FACE_OUTER_BOUND('',#1335,.T.);
#908=FACE_OUTER_BOUND('',#1336,.T.);
#909=FACE_OUTER_BOUND('',#1338,.T.);
#910=FACE_OUTER_BOUND('',#1339,.T.);
#911=FACE_OUTER_BOUND('',#1341,.T.);
#912=FACE_OUTER_BOUND('',#1342,.T.);
#913=FACE_OUTER_BOUND('',#1343,.T.);
#914=FACE_OUTER_BOUND('',#1344,.T.);
#915=FACE_OUTER_BOUND('',#1345,.T.);
#916=FACE_OUTER_BOUND('',#1346,.T.);
#917=FACE_OUTER_BOUND('',#1347,.T.);
#918=FACE_OUTER_BOUND('',#1348,.T.);
#919=FACE_OUTER_BOUND('',#1349,.T.);
#920=FACE_OUTER_BOUND('',#1350,.T.);
#921=FACE_OUTER_BOUND('',#1352,.T.);
#922=FACE_OUTER_BOUND('',#1354,.T.);
#923=FACE_OUTER_BOUND('',#1355,.T.);
#924=FACE_OUTER_BOUND('',#1356,.T.);
#925=FACE_OUTER_BOUND('',#1357,.T.);
#926=FACE_OUTER_BOUND('',#1358,.T.);
#927=FACE_OUTER_BOUND('',#1359,.T.);
#928=FACE_OUTER_BOUND('',#1360,.T.);
#929=FACE_OUTER_BOUND('',#1361,.T.);
#930=FACE_OUTER_BOUND('',#1362,.T.);
#931=FACE_OUTER_BOUND('',#1363,.T.);
#932=FACE_OUTER_BOUND('',#1364,.T.);
#933=FACE_OUTER_BOUND('',#1366,.T.);
#934=FACE_OUTER_BOUND('',#1367,.T.);
#935=FACE_OUTER_BOUND('',#1368,.T.);
#936=FACE_OUTER_BOUND('',#1369,.T.);
#937=FACE_OUTER_BOUND('',#1370,.T.);
#938=FACE_OUTER_BOUND('',#1371,.T.);
#939=FACE_OUTER_BOUND('',#1372,.T.);
#940=FACE_OUTER_BOUND('',#1373,.T.);
#941=FACE_OUTER_BOUND('',#1377,.T.);
#942=FACE_OUTER_BOUND('',#1378,.T.);
#943=FACE_OUTER_BOUND('',#1379,.T.);
#944=FACE_OUTER_BOUND('',#1380,.T.);
#945=FACE_OUTER_BOUND('',#1381,.T.);
#946=FACE_OUTER_BOUND('',#1382,.T.);
#947=FACE_OUTER_BOUND('',#1383,.T.);
#948=FACE_OUTER_BOUND('',#1384,.T.);
#949=FACE_OUTER_BOUND('',#1385,.T.);
#950=FACE_OUTER_BOUND('',#1386,.T.);
#951=FACE_OUTER_BOUND('',#1387,.T.);
#952=FACE_OUTER_BOUND('',#1388,.T.);
#953=FACE_OUTER_BOUND('',#1389,.T.);
#954=FACE_OUTER_BOUND('',#1390,.T.);
#955=FACE_OUTER_BOUND('',#1394,.T.);
#956=FACE_OUTER_BOUND('',#1395,.T.);
#957=FACE_OUTER_BOUND('',#1396,.T.);
#958=FACE_OUTER_BOUND('',#1397,.T.);
#959=FACE_OUTER_BOUND('',#1398,.T.);
#960=FACE_OUTER_BOUND('',#1399,.T.);
#961=FACE_OUTER_BOUND('',#1400,.T.);
#962=FACE_OUTER_BOUND('',#1401,.T.);
#963=FACE_OUTER_BOUND('',#1402,.T.);
#964=FACE_OUTER_BOUND('',#1403,.T.);
#965=FACE_OUTER_BOUND('',#1404,.T.);
#966=FACE_OUTER_BOUND('',#1405,.T.);
#967=FACE_OUTER_BOUND('',#1406,.T.);
#968=FACE_OUTER_BOUND('',#1407,.T.);
#969=FACE_OUTER_BOUND('',#1408,.T.);
#970=FACE_OUTER_BOUND('',#1409,.T.);
#971=FACE_OUTER_BOUND('',#1410,.T.);
#972=FACE_OUTER_BOUND('',#1411,.T.);
#973=FACE_OUTER_BOUND('',#1412,.T.);
#974=FACE_OUTER_BOUND('',#1413,.T.);
#975=FACE_OUTER_BOUND('',#1414,.T.);
#976=FACE_OUTER_BOUND('',#1415,.T.);
#977=FACE_OUTER_BOUND('',#1416,.T.);
#978=FACE_OUTER_BOUND('',#1417,.T.);
#979=FACE_OUTER_BOUND('',#1418,.T.);
#980=FACE_OUTER_BOUND('',#1419,.T.);
#981=FACE_OUTER_BOUND('',#1420,.T.);
#982=FACE_OUTER_BOUND('',#1421,.T.);
#983=FACE_OUTER_BOUND('',#1422,.T.);
#984=FACE_OUTER_BOUND('',#1423,.T.);
#985=FACE_OUTER_BOUND('',#1424,.T.);
#986=FACE_OUTER_BOUND('',#1425,.T.);
#987=FACE_OUTER_BOUND('',#1426,.T.);
#988=FACE_OUTER_BOUND('',#1427,.T.);
#989=FACE_OUTER_BOUND('',#1428,.T.);
#990=FACE_OUTER_BOUND('',#1435,.T.);
#991=FACE_OUTER_BOUND('',#1436,.T.);
#1331=EDGE_LOOP('',(#4949,#4950,#4951,#4952));
#1332=EDGE_LOOP('',(#4953,#4954,#4955,#4956));
#1333=EDGE_LOOP('',(#4957,#4958,#4959,#4960));
#1334=EDGE_LOOP('',(#4961,#4962,#4963,#4964));
#1335=EDGE_LOOP('',(#4965,#4966,#4967,#4968));
#1336=EDGE_LOOP('',(#4969));
#1337=EDGE_LOOP('',(#4970));
#1338=EDGE_LOOP('',(#4971,#4972,#4973,#4974));
#1339=EDGE_LOOP('',(#4975));
#1340=EDGE_LOOP('',(#4976));
#1341=EDGE_LOOP('',(#4977,#4978,#4979,#4980));
#1342=EDGE_LOOP('',(#4981,#4982,#4983,#4984));
#1343=EDGE_LOOP('',(#4985,#4986,#4987,#4988));
#1344=EDGE_LOOP('',(#4989,#4990,#4991,#4992));
#1345=EDGE_LOOP('',(#4993,#4994,#4995,#4996));
#1346=EDGE_LOOP('',(#4997,#4998,#4999,#5000));
#1347=EDGE_LOOP('',(#5001,#5002,#5003,#5004));
#1348=EDGE_LOOP('',(#5005,#5006,#5007,#5008));
#1349=EDGE_LOOP('',(#5009,#5010,#5011,#5012));
#1350=EDGE_LOOP('',(#5013));
#1351=EDGE_LOOP('',(#5014));
#1352=EDGE_LOOP('',(#5015));
#1353=EDGE_LOOP('',(#5016));
#1354=EDGE_LOOP('',(#5017,#5018,#5019,#5020));
#1355=EDGE_LOOP('',(#5021,#5022,#5023,#5024));
#1356=EDGE_LOOP('',(#5025,#5026,#5027,#5028));
#1357=EDGE_LOOP('',(#5029,#5030,#5031,#5032));
#1358=EDGE_LOOP('',(#5033,#5034,#5035,#5036));
#1359=EDGE_LOOP('',(#5037,#5038,#5039,#5040,#5041,#5042));
#1360=EDGE_LOOP('',(#5043,#5044,#5045,#5046,#5047,#5048,#5049,#5050,#5051,
#5052));
#1361=EDGE_LOOP('',(#5053,#5054,#5055,#5056,#5057,#5058,#5059,#5060,#5061,
#5062));
#1362=EDGE_LOOP('',(#5063,#5064,#5065,#5066,#5067,#5068,#5069,#5070,#5071,
#5072));
#1363=EDGE_LOOP('',(#5073,#5074,#5075,#5076,#5077,#5078,#5079,#5080));
#1364=EDGE_LOOP('',(#5081,#5082,#5083,#5084,#5085,#5086,#5087,#5088,#5089,
#5090,#5091,#5092,#5093,#5094,#5095,#5096,#5097,#5098,#5099,#5100,#5101,
#5102,#5103,#5104,#5105,#5106,#5107,#5108,#5109,#5110,#5111,#5112,#5113,
#5114,#5115,#5116,#5117,#5118,#5119,#5120,#5121,#5122));
#1365=EDGE_LOOP('',(#5123,#5124,#5125,#5126,#5127,#5128));
#1366=EDGE_LOOP('',(#5129,#5130,#5131,#5132));
#1367=EDGE_LOOP('',(#5133,#5134,#5135,#5136));
#1368=EDGE_LOOP('',(#5137,#5138,#5139,#5140,#5141,#5142));
#1369=EDGE_LOOP('',(#5143,#5144,#5145,#5146));
#1370=EDGE_LOOP('',(#5147,#5148,#5149,#5150));
#1371=EDGE_LOOP('',(#5151,#5152,#5153,#5154));
#1372=EDGE_LOOP('',(#5155,#5156,#5157,#5158));
#1373=EDGE_LOOP('',(#5159,#5160,#5161,#5162));
#1374=EDGE_LOOP('',(#5163));
#1375=EDGE_LOOP('',(#5164));
#1376=EDGE_LOOP('',(#5165));
#1377=EDGE_LOOP('',(#5166,#5167,#5168,#5169));
#1378=EDGE_LOOP('',(#5170,#5171,#5172,#5173));
#1379=EDGE_LOOP('',(#5174,#5175,#5176,#5177));
#1380=EDGE_LOOP('',(#5178,#5179,#5180,#5181));
#1381=EDGE_LOOP('',(#5182,#5183,#5184,#5185,#5186,#5187,#5188,#5189,#5190,
#5191));
#1382=EDGE_LOOP('',(#5192,#5193,#5194,#5195));
#1383=EDGE_LOOP('',(#5196,#5197,#5198,#5199));
#1384=EDGE_LOOP('',(#5200,#5201,#5202,#5203));
#1385=EDGE_LOOP('',(#5204,#5205,#5206,#5207));
#1386=EDGE_LOOP('',(#5208,#5209,#5210,#5211));
#1387=EDGE_LOOP('',(#5212,#5213,#5214,#5215,#5216,#5217,#5218,#5219,#5220,
#5221));
#1388=EDGE_LOOP('',(#5222,#5223,#5224,#5225));
#1389=EDGE_LOOP('',(#5226,#5227,#5228,#5229));
#1390=EDGE_LOOP('',(#5230,#5231,#5232,#5233));
#1391=EDGE_LOOP('',(#5234));
#1392=EDGE_LOOP('',(#5235));
#1393=EDGE_LOOP('',(#5236));
#1394=EDGE_LOOP('',(#5237,#5238,#5239,#5240));
#1395=EDGE_LOOP('',(#5241,#5242,#5243,#5244));
#1396=EDGE_LOOP('',(#5245,#5246,#5247,#5248,#5249,#5250,#5251,#5252,#5253,
#5254));
#1397=EDGE_LOOP('',(#5255,#5256,#5257,#5258));
#1398=EDGE_LOOP('',(#5259,#5260,#5261,#5262));
#1399=EDGE_LOOP('',(#5263,#5264,#5265,#5266));
#1400=EDGE_LOOP('',(#5267,#5268,#5269,#5270));
#1401=EDGE_LOOP('',(#5271,#5272,#5273,#5274));
#1402=EDGE_LOOP('',(#5275,#5276,#5277));
#1403=EDGE_LOOP('',(#5278,#5279,#5280));
#1404=EDGE_LOOP('',(#5281,#5282,#5283));
#1405=EDGE_LOOP('',(#5284,#5285,#5286,#5287));
#1406=EDGE_LOOP('',(#5288,#5289,#5290,#5291));
#1407=EDGE_LOOP('',(#5292,#5293,#5294));
#1408=EDGE_LOOP('',(#5295,#5296,#5297,#5298));
#1409=EDGE_LOOP('',(#5299,#5300,#5301,#5302));
#1410=EDGE_LOOP('',(#5303,#5304,#5305,#5306));
#1411=EDGE_LOOP('',(#5307,#5308,#5309,#5310));
#1412=EDGE_LOOP('',(#5311,#5312,#5313,#5314));
#1413=EDGE_LOOP('',(#5315,#5316,#5317,#5318));
#1414=EDGE_LOOP('',(#5319,#5320,#5321));
#1415=EDGE_LOOP('',(#5322,#5323,#5324));
#1416=EDGE_LOOP('',(#5325,#5326,#5327));
#1417=EDGE_LOOP('',(#5328,#5329,#5330,#5331));
#1418=EDGE_LOOP('',(#5332,#5333,#5334,#5335));
#1419=EDGE_LOOP('',(#5336,#5337,#5338));
#1420=EDGE_LOOP('',(#5339,#5340,#5341,#5342));
#1421=EDGE_LOOP('',(#5343,#5344,#5345,#5346));
#1422=EDGE_LOOP('',(#5347,#5348,#5349,#5350));
#1423=EDGE_LOOP('',(#5351,#5352,#5353,#5354));
#1424=EDGE_LOOP('',(#5355,#5356,#5357,#5358));
#1425=EDGE_LOOP('',(#5359,#5360,#5361,#5362));
#1426=EDGE_LOOP('',(#5363,#5364,#5365,#5366));
#1427=EDGE_LOOP('',(#5367,#5368,#5369,#5370,#5371,#5372,#5373,#5374));
#1428=EDGE_LOOP('',(#5375,#5376,#5377,#5378));
#1429=EDGE_LOOP('',(#5379));
#1430=EDGE_LOOP('',(#5380));
#1431=EDGE_LOOP('',(#5381));
#1432=EDGE_LOOP('',(#5382));
#1433=EDGE_LOOP('',(#5383));
#1434=EDGE_LOOP('',(#5384));
#1435=EDGE_LOOP('',(#5385,#5386,#5387,#5388));
#1436=EDGE_LOOP('',(#5389,#5390,#5391,#5392));
#1851=LINE('',#9817,#2325);
#1852=LINE('',#9823,#2326);
#1853=LINE('',#9829,#2327);
#1854=LINE('',#9835,#2328);
#1855=LINE('',#9841,#2329);
#1856=LINE('',#9850,#2330);
#1857=LINE('',#9857,#2331);
#1858=LINE('',#9861,#2332);
#1859=LINE('',#9866,#2333);
#1860=LINE('',#9868,#2334);
#1861=LINE('',#9870,#2335);
#1862=LINE('',#9871,#2336);
#1863=LINE('',#9875,#2337);
#1864=LINE('',#9877,#2338);
#1865=LINE('',#9879,#2339);
#1866=LINE('',#9880,#2340);
#1867=LINE('',#9884,#2341);
#1868=LINE('',#9886,#2342);
#1869=LINE('',#9888,#2343);
#1870=LINE('',#9889,#2344);
#1871=LINE('',#9893,#2345);
#1872=LINE('',#9895,#2346);
#1873=LINE('',#9897,#2347);
#1874=LINE('',#9898,#2348);
#1875=LINE('',#9902,#2349);
#1876=LINE('',#9904,#2350);
#1877=LINE('',#9906,#2351);
#1878=LINE('',#9907,#2352);
#1879=LINE('',#9911,#2353);
#1880=LINE('',#9913,#2354);
#1881=LINE('',#9915,#2355);
#1882=LINE('',#9916,#2356);
#1883=LINE('',#9920,#2357);
#1884=LINE('',#9922,#2358);
#1885=LINE('',#9924,#2359);
#1886=LINE('',#9925,#2360);
#1887=LINE('',#9933,#2361);
#1888=LINE('',#9934,#2362);
#1889=LINE('',#9936,#2363);
#1890=LINE('',#9937,#2364);
#1891=LINE('',#9939,#2365);
#1892=LINE('',#9940,#2366);
#1893=LINE('',#9943,#2367);
#1894=LINE('',#9945,#2368);
#1895=LINE('',#9946,#2369);
#1896=LINE('',#9949,#2370);
#1897=LINE('',#9951,#2371);
#1898=LINE('',#9952,#2372);
#1899=LINE('',#9956,#2373);
#1900=LINE('',#9994,#2374);
#1901=LINE('',#10032,#2375);
#1902=LINE('',#10070,#2376);
#1903=LINE('',#10107,#2377);
#1904=LINE('',#10110,#2378);
#1905=LINE('',#10148,#2379);
#1906=LINE('',#10185,#2380);
#1907=LINE('',#10188,#2381);
#1908=LINE('',#10226,#2382);
#1909=LINE('',#10263,#2383);
#1910=LINE('',#10266,#2384);
#1911=LINE('',#10273,#2385);
#1912=LINE('',#10279,#2386);
#1913=LINE('',#10296,#2387);
#1914=LINE('',#10305,#2388);
#1915=LINE('',#10311,#2389);
#1916=LINE('',#10346,#2390);
#1917=LINE('',#10417,#2391);
#1918=LINE('',#10487,#2392);
#1919=LINE('',#10522,#2393);
#1920=LINE('',#10528,#2394);
#1921=LINE('',#10537,#2395);
#1922=LINE('',#10571,#2396);
#1923=LINE('',#10603,#2397);
#1924=LINE('',#10607,#2398);
#1925=LINE('',#10611,#2399);
#1926=LINE('',#10657,#2400);
#1927=LINE('',#10792,#2401);
#1928=LINE('',#10896,#2402);
#1929=LINE('',#11059,#2403);
#1930=LINE('',#11222,#2404);
#1931=LINE('',#11311,#2405);
#1932=LINE('',#11399,#2406);
#1933=LINE('',#11511,#2407);
#1934=LINE('',#11512,#2408);
#1935=LINE('',#11549,#2409);
#1936=LINE('',#11550,#2410);
#2325=VECTOR('',#8269,0.15);
#2326=VECTOR('',#8276,0.15);
#2327=VECTOR('',#8283,0.15);
#2328=VECTOR('',#8290,0.15);
#2329=VECTOR('',#8297,0.3);
#2330=VECTOR('',#8308,0.3);
#2331=VECTOR('',#8317,0.17);
#2332=VECTOR('',#8322,0.17);
#2333=VECTOR('',#8327,1.);
#2334=VECTOR('',#8328,1.);
#2335=VECTOR('',#8329,1.);
#2336=VECTOR('',#8330,1.);
#2337=VECTOR('',#8333,1.);
#2338=VECTOR('',#8334,1.);
#2339=VECTOR('',#8335,1.);
#2340=VECTOR('',#8336,1.);
#2341=VECTOR('',#8339,1.);
#2342=VECTOR('',#8340,1.);
#2343=VECTOR('',#8341,1.);
#2344=VECTOR('',#8342,1.);
#2345=VECTOR('',#8345,1.);
#2346=VECTOR('',#8346,1.);
#2347=VECTOR('',#8347,1.);
#2348=VECTOR('',#8348,1.);
#2349=VECTOR('',#8351,1.);
#2350=VECTOR('',#8352,1.);
#2351=VECTOR('',#8353,1.);
#2352=VECTOR('',#8354,1.);
#2353=VECTOR('',#8357,1.);
#2354=VECTOR('',#8358,1.);
#2355=VECTOR('',#8359,1.);
#2356=VECTOR('',#8360,1.);
#2357=VECTOR('',#8363,1.);
#2358=VECTOR('',#8364,1.);
#2359=VECTOR('',#8365,1.);
#2360=VECTOR('',#8366,1.);
#2361=VECTOR('',#8377,1.);
#2362=VECTOR('',#8378,1.);
#2363=VECTOR('',#8381,1.);
#2364=VECTOR('',#8382,1.);
#2365=VECTOR('',#8385,1.);
#2366=VECTOR('',#8386,1.);
#2367=VECTOR('',#8389,1.);
#2368=VECTOR('',#8390,1.);
#2369=VECTOR('',#8391,1.);
#2370=VECTOR('',#8394,1.);
#2371=VECTOR('',#8395,1.);
#2372=VECTOR('',#8396,1.);
#2373=VECTOR('',#8399,1.);
#2374=VECTOR('',#8400,1.);
#2375=VECTOR('',#8403,1.);
#2376=VECTOR('',#8404,1.);
#2377=VECTOR('',#8405,1.);
#2378=VECTOR('',#8408,1.);
#2379=VECTOR('',#8409,1.);
#2380=VECTOR('',#8410,1.);
#2381=VECTOR('',#8413,1.);
#2382=VECTOR('',#8414,1.);
#2383=VECTOR('',#8415,1.);
#2384=VECTOR('',#8418,1.);
#2385=VECTOR('',#8419,1.);
#2386=VECTOR('',#8420,1.);
#2387=VECTOR('',#8423,1.);
#2388=VECTOR('',#8424,1.);
#2389=VECTOR('',#8425,1.);
#2390=VECTOR('',#8426,1.);
#2391=VECTOR('',#8427,1.);
#2392=VECTOR('',#8428,1.);
#2393=VECTOR('',#8429,1.);
#2394=VECTOR('',#8430,1.);
#2395=VECTOR('',#8431,1.);
#2396=VECTOR('',#8432,1.);
#2397=VECTOR('',#8433,1.);
#2398=VECTOR('',#8438,0.4);
#2399=VECTOR('',#8443,0.4);
#2400=VECTOR('',#8446,1.);
#2401=VECTOR('',#8453,1.);
#2402=VECTOR('',#8456,1.);
#2403=VECTOR('',#8461,1.);
#2404=VECTOR('',#8466,1.);
#2405=VECTOR('',#8471,1.);
#2406=VECTOR('',#8504,1.);
#2407=VECTOR('',#8533,1.);
#2408=VECTOR('',#8534,1.);
#2409=VECTOR('',#8545,1.);
#2410=VECTOR('',#8546,1.);
#2719=CIRCLE('',#7425,0.15);
#2720=CIRCLE('',#7426,0.15);
#2721=CIRCLE('',#7428,0.15);
#2722=CIRCLE('',#7429,0.15);
#2723=CIRCLE('',#7431,0.15);
#2724=CIRCLE('',#7432,0.15);
#2725=CIRCLE('',#7434,0.15);
#2726=CIRCLE('',#7435,0.15);
#2727=CIRCLE('',#7437,0.3);
#2728=CIRCLE('',#7438,0.3);
#2729=CIRCLE('',#7440,0.17);
#2730=CIRCLE('',#7442,0.3);
#2731=CIRCLE('',#7443,0.3);
#2732=CIRCLE('',#7445,0.17);
#2733=CIRCLE('',#7447,0.17);
#2734=CIRCLE('',#7449,0.17);
#2735=CIRCLE('',#7458,0.4);
#2736=CIRCLE('',#7460,0.4);
#2737=CIRCLE('',#7473,0.4);
#2738=CIRCLE('',#7475,0.4);
#2739=CIRCLE('',#7477,0.1);
#2740=CIRCLE('',#7485,0.0999999999999994);
#2741=CIRCLE('',#7487,0.0999999999999999);
#2742=CIRCLE('',#7489,0.1);
#2743=CIRCLE('',#7490,0.1);
#2744=CIRCLE('',#7492,0.100000000000001);
#2745=CIRCLE('',#7493,0.100000000000001);
#2746=CIRCLE('',#7494,0.100000000000002);
#2747=CIRCLE('',#7496,0.0999999999999995);
#2748=CIRCLE('',#7497,0.0999999999999991);
#2749=CIRCLE('',#7500,0.100000000000001);
#2750=CIRCLE('',#7501,0.1);
#2751=CIRCLE('',#7505,0.3);
#2752=CIRCLE('',#7506,0.3);
#2753=CIRCLE('',#7507,0.3);
#2754=CIRCLE('',#7509,0.3);
#2755=CIRCLE('',#7510,0.300000000000002);
#2756=CIRCLE('',#7511,0.3);
#2757=CIRCLE('',#7513,0.3);
#2758=CIRCLE('',#7514,0.299999999999999);
#2759=CIRCLE('',#7515,0.3);
#2760=CIRCLE('',#7518,0.300000000000001);
#2761=CIRCLE('',#7519,0.3);
#2762=CIRCLE('',#7520,0.3);
#2979=VERTEX_POINT('',#9814);
#2980=VERTEX_POINT('',#9816);
#2981=VERTEX_POINT('',#9820);
#2982=VERTEX_POINT('',#9822);
#2983=VERTEX_POINT('',#9826);
#2984=VERTEX_POINT('',#9828);
#2985=VERTEX_POINT('',#9832);
#2986=VERTEX_POINT('',#9834);
#2987=VERTEX_POINT('',#9838);
#2988=VERTEX_POINT('',#9840);
#2989=VERTEX_POINT('',#9844);
#2990=VERTEX_POINT('',#9847);
#2991=VERTEX_POINT('',#9849);
#2992=VERTEX_POINT('',#9853);
#2993=VERTEX_POINT('',#9856);
#2994=VERTEX_POINT('',#9860);
#2995=VERTEX_POINT('',#9864);
#2996=VERTEX_POINT('',#9865);
#2997=VERTEX_POINT('',#9867);
#2998=VERTEX_POINT('',#9869);
#2999=VERTEX_POINT('',#9873);
#3000=VERTEX_POINT('',#9874);
#3001=VERTEX_POINT('',#9876);
#3002=VERTEX_POINT('',#9878);
#3003=VERTEX_POINT('',#9882);
#3004=VERTEX_POINT('',#9883);
#3005=VERTEX_POINT('',#9885);
#3006=VERTEX_POINT('',#9887);
#3007=VERTEX_POINT('',#9891);
#3008=VERTEX_POINT('',#9892);
#3009=VERTEX_POINT('',#9894);
#3010=VERTEX_POINT('',#9896);
#3011=VERTEX_POINT('',#9900);
#3012=VERTEX_POINT('',#9901);
#3013=VERTEX_POINT('',#9903);
#3014=VERTEX_POINT('',#9905);
#3015=VERTEX_POINT('',#9909);
#3016=VERTEX_POINT('',#9910);
#3017=VERTEX_POINT('',#9912);
#3018=VERTEX_POINT('',#9914);
#3019=VERTEX_POINT('',#9918);
#3020=VERTEX_POINT('',#9919);
#3021=VERTEX_POINT('',#9921);
#3022=VERTEX_POINT('',#9923);
#3023=VERTEX_POINT('',#9927);
#3024=VERTEX_POINT('',#9930);
#3025=VERTEX_POINT('',#9942);
#3026=VERTEX_POINT('',#9944);
#3027=VERTEX_POINT('',#9948);
#3028=VERTEX_POINT('',#9950);
#3029=VERTEX_POINT('',#9954);
#3030=VERTEX_POINT('',#9955);
#3031=VERTEX_POINT('',#9957);
#3032=VERTEX_POINT('',#9964);
#3033=VERTEX_POINT('',#9993);
#3034=VERTEX_POINT('',#9995);
#3035=VERTEX_POINT('',#10031);
#3036=VERTEX_POINT('',#10033);
#3037=VERTEX_POINT('',#10040);
#3038=VERTEX_POINT('',#10069);
#3039=VERTEX_POINT('',#10071);
#3040=VERTEX_POINT('',#10100);
#3041=VERTEX_POINT('',#10109);
#3042=VERTEX_POINT('',#10111);
#3043=VERTEX_POINT('',#10118);
#3044=VERTEX_POINT('',#10147);
#3045=VERTEX_POINT('',#10149);
#3046=VERTEX_POINT('',#10178);
#3047=VERTEX_POINT('',#10187);
#3048=VERTEX_POINT('',#10189);
#3049=VERTEX_POINT('',#10196);
#3050=VERTEX_POINT('',#10225);
#3051=VERTEX_POINT('',#10227);
#3052=VERTEX_POINT('',#10256);
#3053=VERTEX_POINT('',#10265);
#3054=VERTEX_POINT('',#10267);
#3055=VERTEX_POINT('',#10272);
#3056=VERTEX_POINT('',#10274);
#3057=VERTEX_POINT('',#10295);
#3058=VERTEX_POINT('',#10304);
#3059=VERTEX_POINT('',#10310);
#3060=VERTEX_POINT('',#10312);
#3061=VERTEX_POINT('',#10345);
#3062=VERTEX_POINT('',#10347);
#3063=VERTEX_POINT('',#10379);
#3064=VERTEX_POINT('',#10384);
#3065=VERTEX_POINT('',#10416);
#3066=VERTEX_POINT('',#10418);
#3067=VERTEX_POINT('',#10450);
#3068=VERTEX_POINT('',#10455);
#3069=VERTEX_POINT('',#10488);
#3070=VERTEX_POINT('',#10517);
#3071=VERTEX_POINT('',#10523);
#3072=VERTEX_POINT('',#10529);
#3073=VERTEX_POINT('',#10538);
#3074=VERTEX_POINT('',#10539);
#3075=VERTEX_POINT('',#10544);
#3076=VERTEX_POINT('',#10570);
#3077=VERTEX_POINT('',#10572);
#3078=VERTEX_POINT('',#10598);
#3079=VERTEX_POINT('',#10605);
#3080=VERTEX_POINT('',#10609);
#3081=VERTEX_POINT('',#10613);
#3082=VERTEX_POINT('',#10620);
#3083=VERTEX_POINT('',#10627);
#3084=VERTEX_POINT('',#10656);
#3085=VERTEX_POINT('',#10722);
#3086=VERTEX_POINT('',#10775);
#3087=VERTEX_POINT('',#10787);
#3088=VERTEX_POINT('',#10849);
#3089=VERTEX_POINT('',#10859);
#3090=VERTEX_POINT('',#10866);
#3091=VERTEX_POINT('',#10895);
#3092=VERTEX_POINT('',#10897);
#3093=VERTEX_POINT('',#11022);
#3094=VERTEX_POINT('',#11029);
#3095=VERTEX_POINT('',#11058);
#3096=VERTEX_POINT('',#11060);
#3097=VERTEX_POINT('',#11185);
#3098=VERTEX_POINT('',#11192);
#3099=VERTEX_POINT('',#11221);
#3100=VERTEX_POINT('',#11223);
#3101=VERTEX_POINT('',#11274);
#3102=VERTEX_POINT('',#11303);
#3103=VERTEX_POINT('',#11310);
#3104=VERTEX_POINT('',#11332);
#3105=VERTEX_POINT('',#11367);
#3106=VERTEX_POINT('',#11395);
#3107=VERTEX_POINT('',#11490);
#3108=VERTEX_POINT('',#11491);
#3109=VERTEX_POINT('',#11493);
#3110=VERTEX_POINT('',#11497);
#3111=VERTEX_POINT('',#11498);
#3112=VERTEX_POINT('',#11500);
#3113=VERTEX_POINT('',#11504);
#3114=VERTEX_POINT('',#11505);
#3115=VERTEX_POINT('',#11507);
#3116=VERTEX_POINT('',#11542);
#3117=VERTEX_POINT('',#11543);
#3118=VERTEX_POINT('',#11545);
#3715=EDGE_CURVE('',#2979,#2979,#2719,.T.);
#3716=EDGE_CURVE('',#2979,#2980,#1851,.T.);
#3717=EDGE_CURVE('',#2980,#2980,#2720,.T.);
#3718=EDGE_CURVE('',#2981,#2981,#2721,.T.);
#3719=EDGE_CURVE('',#2981,#2982,#1852,.T.);
#3720=EDGE_CURVE('',#2982,#2982,#2722,.T.);
#3721=EDGE_CURVE('',#2983,#2983,#2723,.T.);
#3722=EDGE_CURVE('',#2983,#2984,#1853,.T.);
#3723=EDGE_CURVE('',#2984,#2984,#2724,.T.);
#3724=EDGE_CURVE('',#2985,#2985,#2725,.T.);
#3725=EDGE_CURVE('',#2985,#2986,#1854,.T.);
#3726=EDGE_CURVE('',#2986,#2986,#2726,.T.);
#3727=EDGE_CURVE('',#2987,#2987,#2727,.T.);
#3728=EDGE_CURVE('',#2987,#2988,#1855,.T.);
#3729=EDGE_CURVE('',#2988,#2988,#2728,.T.);
#3730=EDGE_CURVE('',#2989,#2989,#2729,.T.);
#3731=EDGE_CURVE('',#2990,#2990,#2730,.T.);
#3732=EDGE_CURVE('',#2990,#2991,#1856,.T.);
#3733=EDGE_CURVE('',#2991,#2991,#2731,.T.);
#3734=EDGE_CURVE('',#2992,#2992,#2732,.T.);
#3735=EDGE_CURVE('',#2989,#2993,#1857,.T.);
#3736=EDGE_CURVE('',#2993,#2993,#2733,.T.);
#3737=EDGE_CURVE('',#2992,#2994,#1858,.T.);
#3738=EDGE_CURVE('',#2994,#2994,#2734,.T.);
#3739=EDGE_CURVE('',#2995,#2996,#1859,.T.);
#3740=EDGE_CURVE('',#2997,#2995,#1860,.T.);
#3741=EDGE_CURVE('',#2998,#2997,#1861,.T.);
#3742=EDGE_CURVE('',#2998,#2996,#1862,.T.);
#3743=EDGE_CURVE('',#2999,#3000,#1863,.T.);
#3744=EDGE_CURVE('',#2999,#3001,#1864,.T.);
#3745=EDGE_CURVE('',#3002,#3001,#1865,.T.);
#3746=EDGE_CURVE('',#3000,#3002,#1866,.T.);
#3747=EDGE_CURVE('',#3003,#3004,#1867,.T.);
#3748=EDGE_CURVE('',#3003,#3005,#1868,.T.);
#3749=EDGE_CURVE('',#3006,#3005,#1869,.T.);
#3750=EDGE_CURVE('',#3004,#3006,#1870,.T.);
#3751=EDGE_CURVE('',#3007,#3008,#1871,.T.);
#3752=EDGE_CURVE('',#3007,#3009,#1872,.T.);
#3753=EDGE_CURVE('',#3010,#3009,#1873,.T.);
#3754=EDGE_CURVE('',#3008,#3010,#1874,.T.);
#3755=EDGE_CURVE('',#3011,#3012,#1875,.T.);
#3756=EDGE_CURVE('',#3011,#3013,#1876,.T.);
#3757=EDGE_CURVE('',#3014,#3013,#1877,.T.);
#3758=EDGE_CURVE('',#3012,#3014,#1878,.T.);
#3759=EDGE_CURVE('',#3015,#3016,#1879,.T.);
#3760=EDGE_CURVE('',#3017,#3015,#1880,.T.);
#3761=EDGE_CURVE('',#3018,#3017,#1881,.T.);
#3762=EDGE_CURVE('',#3018,#3016,#1882,.T.);
#3763=EDGE_CURVE('',#3019,#3020,#1883,.T.);
#3764=EDGE_CURVE('',#3021,#3019,#1884,.T.);
#3765=EDGE_CURVE('',#3022,#3021,#1885,.T.);
#3766=EDGE_CURVE('',#3022,#3020,#1886,.T.);
#3767=EDGE_CURVE('',#3023,#3023,#2735,.T.);
#3768=EDGE_CURVE('',#3024,#3024,#2736,.T.);
#3769=EDGE_CURVE('',#2996,#3011,#1887,.T.);
#3770=EDGE_CURVE('',#3013,#2998,#1888,.T.);
#3771=EDGE_CURVE('',#3016,#2999,#1889,.T.);
#3772=EDGE_CURVE('',#3001,#3018,#1890,.T.);
#3773=EDGE_CURVE('',#3020,#3003,#1891,.T.);
#3774=EDGE_CURVE('',#3005,#3022,#1892,.T.);
#3775=EDGE_CURVE('',#3025,#3007,#1893,.T.);
#3776=EDGE_CURVE('',#3026,#3025,#1894,.T.);
#3777=EDGE_CURVE('',#3009,#3026,#1895,.T.);
#3778=EDGE_CURVE('',#3027,#3025,#1896,.T.);
#3779=EDGE_CURVE('',#3028,#3027,#1897,.T.);
#3780=EDGE_CURVE('',#3026,#3028,#1898,.T.);
#3781=EDGE_CURVE('',#3029,#3030,#1899,.T.);
#3782=EDGE_CURVE('',#3031,#3030,#172,.T.);
#3783=EDGE_CURVE('',#3032,#3031,#173,.T.);
#3784=EDGE_CURVE('',#3033,#3032,#1900,.T.);
#3785=EDGE_CURVE('',#3034,#3033,#174,.T.);
#3786=EDGE_CURVE('',#3029,#3034,#175,.T.);
#3787=EDGE_CURVE('',#3028,#3035,#1901,.T.);
#3788=EDGE_CURVE('',#3036,#3035,#176,.T.);
#3789=EDGE_CURVE('',#3037,#3036,#177,.T.);
#3790=EDGE_CURVE('',#3038,#3037,#1902,.T.);
#3791=EDGE_CURVE('',#3039,#3038,#178,.T.);
#3792=EDGE_CURVE('',#3040,#3039,#179,.T.);
#3793=EDGE_CURVE('',#3040,#3010,#1903,.T.);
#3794=EDGE_CURVE('',#3021,#3041,#1904,.T.);
#3795=EDGE_CURVE('',#3042,#3041,#180,.T.);
#3796=EDGE_CURVE('',#3043,#3042,#181,.T.);
#3797=EDGE_CURVE('',#3044,#3043,#1905,.T.);
#3798=EDGE_CURVE('',#3045,#3044,#182,.T.);
#3799=EDGE_CURVE('',#3046,#3045,#183,.T.);
#3800=EDGE_CURVE('',#3046,#3006,#1906,.T.);
#3801=EDGE_CURVE('',#3017,#3047,#1907,.T.);
#3802=EDGE_CURVE('',#3048,#3047,#184,.T.);
#3803=EDGE_CURVE('',#3049,#3048,#185,.T.);
#3804=EDGE_CURVE('',#3050,#3049,#1908,.T.);
#3805=EDGE_CURVE('',#3051,#3050,#186,.T.);
#3806=EDGE_CURVE('',#3052,#3051,#187,.T.);
#3807=EDGE_CURVE('',#3052,#3002,#1909,.T.);
#3808=EDGE_CURVE('',#3053,#3012,#1910,.T.);
#3809=EDGE_CURVE('',#3053,#3054,#188,.T.);
#3810=EDGE_CURVE('',#3054,#3055,#1911,.T.);
#3811=EDGE_CURVE('',#3055,#3056,#189,.T.);
#3812=EDGE_CURVE('',#2995,#3056,#1912,.T.);
#3813=EDGE_CURVE('',#3040,#3030,#190,.T.);
#3814=EDGE_CURVE('',#3029,#3035,#191,.T.);
#3815=EDGE_CURVE('',#3057,#3027,#1913,.T.);
#3816=EDGE_CURVE('',#3057,#3041,#192,.T.);
#3817=EDGE_CURVE('',#3058,#3019,#1914,.T.);
#3818=EDGE_CURVE('',#3058,#3047,#193,.T.);
#3819=EDGE_CURVE('',#3059,#3015,#1915,.T.);
#3820=EDGE_CURVE('',#3059,#3060,#194,.T.);
#3821=EDGE_CURVE('',#3060,#3053,#195,.T.);
#3822=EDGE_CURVE('',#3014,#3061,#1916,.T.);
#3823=EDGE_CURVE('',#3062,#3061,#196,.T.);
#3824=EDGE_CURVE('',#3062,#3063,#197,.T.);
#3825=EDGE_CURVE('',#3064,#3063,#198,.T.);
#3826=EDGE_CURVE('',#3064,#3065,#1917,.T.);
#3827=EDGE_CURVE('',#3066,#3065,#199,.T.);
#3828=EDGE_CURVE('',#3066,#3067,#200,.T.);
#3829=EDGE_CURVE('',#3068,#3067,#201,.T.);
#3830=EDGE_CURVE('',#3068,#2997,#1918,.T.);
#3831=EDGE_CURVE('',#3056,#3069,#202,.T.);
#3832=EDGE_CURVE('',#3069,#3070,#203,.T.);
#3833=EDGE_CURVE('',#3000,#3070,#1919,.T.);
#3834=EDGE_CURVE('',#3052,#3071,#204,.T.);
#3835=EDGE_CURVE('',#3004,#3071,#1920,.T.);
#3836=EDGE_CURVE('',#3046,#3072,#205,.T.);
#3837=EDGE_CURVE('',#3008,#3072,#1921,.T.);
#3838=EDGE_CURVE('',#3073,#3074,#206,.T.);
#3839=EDGE_CURVE('',#3074,#3075,#207,.T.);
#3840=EDGE_CURVE('',#3075,#3076,#1922,.T.);
#3841=EDGE_CURVE('',#3076,#3077,#208,.T.);
#3842=EDGE_CURVE('',#3077,#3078,#209,.T.);
#3843=EDGE_CURVE('',#3073,#3078,#1923,.T.);
#3844=EDGE_CURVE('',#3079,#3079,#2737,.T.);
#3845=EDGE_CURVE('',#3079,#3024,#1924,.T.);
#3846=EDGE_CURVE('',#3080,#3080,#2738,.T.);
#3847=EDGE_CURVE('',#3080,#3023,#1925,.T.);
#3848=EDGE_CURVE('',#3073,#3081,#210,.T.);
#3849=EDGE_CURVE('',#3082,#3078,#211,.T.);
#3850=EDGE_CURVE('',#3083,#3082,#212,.T.);
#3851=EDGE_CURVE('',#3084,#3083,#1926,.T.);
#3852=EDGE_CURVE('',#3081,#3084,#213,.T.);
#3853=EDGE_CURVE('',#3039,#3031,#214,.T.);
#3854=EDGE_CURVE('',#3081,#3085,#215,.T.);
#3855=EDGE_CURVE('',#3085,#3074,#216,.T.);
#3856=EDGE_CURVE('',#3032,#3038,#217,.T.);
#3857=EDGE_CURVE('',#3086,#3084,#218,.T.);
#3858=EDGE_CURVE('',#3085,#3086,#2739,.F.);
#3859=EDGE_CURVE('',#3037,#3033,#219,.T.);
#3860=EDGE_CURVE('',#3083,#3087,#220,.T.);
#3861=EDGE_CURVE('',#3087,#3086,#1927,.T.);
#3862=EDGE_CURVE('',#3034,#3036,#221,.T.);
#3863=EDGE_CURVE('',#3077,#3088,#222,.T.);
#3864=EDGE_CURVE('',#3088,#3082,#223,.T.);
#3865=EDGE_CURVE('',#3089,#3072,#224,.T.);
#3866=EDGE_CURVE('',#3090,#3089,#225,.T.);
#3867=EDGE_CURVE('',#3091,#3090,#1928,.T.);
#3868=EDGE_CURVE('',#3092,#3091,#226,.T.);
#3869=EDGE_CURVE('',#3057,#3092,#227,.T.);
#3870=EDGE_CURVE('',#3045,#3089,#228,.T.);
#3871=EDGE_CURVE('',#3090,#3044,#229,.T.);
#3872=EDGE_CURVE('',#3043,#3091,#230,.T.);
#3873=EDGE_CURVE('',#3092,#3042,#231,.T.);
#3874=EDGE_CURVE('',#3093,#3071,#232,.T.);
#3875=EDGE_CURVE('',#3094,#3093,#233,.T.);
#3876=EDGE_CURVE('',#3095,#3094,#1929,.T.);
#3877=EDGE_CURVE('',#3096,#3095,#234,.T.);
#3878=EDGE_CURVE('',#3058,#3096,#235,.T.);
#3879=EDGE_CURVE('',#3051,#3093,#236,.T.);
#3880=EDGE_CURVE('',#3094,#3050,#237,.T.);
#3881=EDGE_CURVE('',#3049,#3095,#238,.T.);
#3882=EDGE_CURVE('',#3096,#3048,#239,.T.);
#3883=EDGE_CURVE('',#3097,#3070,#240,.T.);
#3884=EDGE_CURVE('',#3098,#3097,#241,.T.);
#3885=EDGE_CURVE('',#3099,#3098,#1930,.T.);
#3886=EDGE_CURVE('',#3100,#3099,#242,.T.);
#3887=EDGE_CURVE('',#3059,#3100,#243,.T.);
#3888=EDGE_CURVE('',#3069,#3101,#244,.T.);
#3889=EDGE_CURVE('',#3101,#3097,#245,.T.);
#3890=EDGE_CURVE('',#3102,#3101,#2740,.F.);
#3891=EDGE_CURVE('',#3098,#3102,#246,.T.);
#3892=EDGE_CURVE('',#3102,#3103,#1931,.T.);
#3893=EDGE_CURVE('',#3103,#3099,#247,.T.);
#3894=EDGE_CURVE('',#3100,#3104,#248,.T.);
#3895=EDGE_CURVE('',#3104,#3060,#249,.T.);
#3896=EDGE_CURVE('',#3104,#3103,#2741,.F.);
#3897=EDGE_CURVE('',#3103,#3054,#2742,.F.);
#3898=EDGE_CURVE('',#3054,#3104,#2743,.F.);
#3899=EDGE_CURVE('',#3087,#3088,#2744,.F.);
#3900=EDGE_CURVE('',#3088,#3105,#2745,.F.);
#3901=EDGE_CURVE('',#3105,#3087,#2746,.F.);
#3902=EDGE_CURVE('',#3101,#3055,#2747,.F.);
#3903=EDGE_CURVE('',#3055,#3102,#2748,.F.);
#3904=EDGE_CURVE('',#3106,#3085,#2749,.F.);
#3905=EDGE_CURVE('',#3086,#3106,#2750,.F.);
#3906=EDGE_CURVE('',#3106,#3105,#1932,.T.);
#3907=EDGE_CURVE('',#3075,#3106,#250,.T.);
#3908=EDGE_CURVE('',#3105,#3076,#251,.T.);
#3909=EDGE_CURVE('',#3107,#3108,#2751,.F.);
#3910=EDGE_CURVE('',#3109,#3107,#2752,.F.);
#3911=EDGE_CURVE('',#3108,#3109,#2753,.F.);
#3912=EDGE_CURVE('',#3110,#3111,#2754,.F.);
#3913=EDGE_CURVE('',#3112,#3110,#2755,.F.);
#3914=EDGE_CURVE('',#3111,#3112,#2756,.F.);
#3915=EDGE_CURVE('',#3113,#3114,#2757,.F.);
#3916=EDGE_CURVE('',#3115,#3113,#2758,.F.);
#3917=EDGE_CURVE('',#3114,#3115,#2759,.F.);
#3918=EDGE_CURVE('',#3108,#3115,#1933,.T.);
#3919=EDGE_CURVE('',#3113,#3107,#1934,.T.);
#3920=EDGE_CURVE('',#3067,#3114,#252,.T.);
#3921=EDGE_CURVE('',#3115,#3068,#253,.T.);
#3922=EDGE_CURVE('',#3116,#3117,#2760,.F.);
#3923=EDGE_CURVE('',#3118,#3116,#2761,.F.);
#3924=EDGE_CURVE('',#3117,#3118,#2762,.F.);
#3925=EDGE_CURVE('',#3116,#3112,#1935,.T.);
#3926=EDGE_CURVE('',#3110,#3118,#1936,.T.);
#3927=EDGE_CURVE('',#3114,#3117,#254,.T.);
#3928=EDGE_CURVE('',#3118,#3113,#255,.T.);
#3929=EDGE_CURVE('',#3065,#3116,#256,.T.);
#3930=EDGE_CURVE('',#3117,#3066,#257,.T.);
#3931=EDGE_CURVE('',#3063,#3111,#258,.T.);
#3932=EDGE_CURVE('',#3112,#3064,#259,.T.);
#3933=EDGE_CURVE('',#3111,#3109,#260,.T.);
#3934=EDGE_CURVE('',#3107,#3110,#261,.T.);
#3935=EDGE_CURVE('',#3061,#3108,#262,.T.);
#3936=EDGE_CURVE('',#3109,#3062,#263,.T.);
#4949=ORIENTED_EDGE('',*,*,#3715,.F.);
#4950=ORIENTED_EDGE('',*,*,#3716,.T.);
#4951=ORIENTED_EDGE('',*,*,#3717,.F.);
#4952=ORIENTED_EDGE('',*,*,#3716,.F.);
#4953=ORIENTED_EDGE('',*,*,#3718,.F.);
#4954=ORIENTED_EDGE('',*,*,#3719,.T.);
#4955=ORIENTED_EDGE('',*,*,#3720,.F.);
#4956=ORIENTED_EDGE('',*,*,#3719,.F.);
#4957=ORIENTED_EDGE('',*,*,#3721,.F.);
#4958=ORIENTED_EDGE('',*,*,#3722,.T.);
#4959=ORIENTED_EDGE('',*,*,#3723,.F.);
#4960=ORIENTED_EDGE('',*,*,#3722,.F.);
#4961=ORIENTED_EDGE('',*,*,#3724,.F.);
#4962=ORIENTED_EDGE('',*,*,#3725,.T.);
#4963=ORIENTED_EDGE('',*,*,#3726,.F.);
#4964=ORIENTED_EDGE('',*,*,#3725,.F.);
#4965=ORIENTED_EDGE('',*,*,#3727,.F.);
#4966=ORIENTED_EDGE('',*,*,#3728,.T.);
#4967=ORIENTED_EDGE('',*,*,#3729,.T.);
#4968=ORIENTED_EDGE('',*,*,#3728,.F.);
#4969=ORIENTED_EDGE('',*,*,#3729,.F.);
#4970=ORIENTED_EDGE('',*,*,#3730,.F.);
#4971=ORIENTED_EDGE('',*,*,#3731,.F.);
#4972=ORIENTED_EDGE('',*,*,#3732,.T.);
#4973=ORIENTED_EDGE('',*,*,#3733,.T.);
#4974=ORIENTED_EDGE('',*,*,#3732,.F.);
#4975=ORIENTED_EDGE('',*,*,#3733,.F.);
#4976=ORIENTED_EDGE('',*,*,#3734,.F.);
#4977=ORIENTED_EDGE('',*,*,#3730,.T.);
#4978=ORIENTED_EDGE('',*,*,#3735,.T.);
#4979=ORIENTED_EDGE('',*,*,#3736,.F.);
#4980=ORIENTED_EDGE('',*,*,#3735,.F.);
#4981=ORIENTED_EDGE('',*,*,#3734,.T.);
#4982=ORIENTED_EDGE('',*,*,#3737,.T.);
#4983=ORIENTED_EDGE('',*,*,#3738,.F.);
#4984=ORIENTED_EDGE('',*,*,#3737,.F.);
#4985=ORIENTED_EDGE('',*,*,#3739,.F.);
#4986=ORIENTED_EDGE('',*,*,#3740,.F.);
#4987=ORIENTED_EDGE('',*,*,#3741,.F.);
#4988=ORIENTED_EDGE('',*,*,#3742,.T.);
#4989=ORIENTED_EDGE('',*,*,#3743,.F.);
#4990=ORIENTED_EDGE('',*,*,#3744,.T.);
#4991=ORIENTED_EDGE('',*,*,#3745,.F.);
#4992=ORIENTED_EDGE('',*,*,#3746,.F.);
#4993=ORIENTED_EDGE('',*,*,#3747,.F.);
#4994=ORIENTED_EDGE('',*,*,#3748,.T.);
#4995=ORIENTED_EDGE('',*,*,#3749,.F.);
#4996=ORIENTED_EDGE('',*,*,#3750,.F.);
#4997=ORIENTED_EDGE('',*,*,#3751,.F.);
#4998=ORIENTED_EDGE('',*,*,#3752,.T.);
#4999=ORIENTED_EDGE('',*,*,#3753,.F.);
#5000=ORIENTED_EDGE('',*,*,#3754,.F.);
#5001=ORIENTED_EDGE('',*,*,#3755,.F.);
#5002=ORIENTED_EDGE('',*,*,#3756,.T.);
#5003=ORIENTED_EDGE('',*,*,#3757,.F.);
#5004=ORIENTED_EDGE('',*,*,#3758,.F.);
#5005=ORIENTED_EDGE('',*,*,#3759,.F.);
#5006=ORIENTED_EDGE('',*,*,#3760,.F.);
#5007=ORIENTED_EDGE('',*,*,#3761,.F.);
#5008=ORIENTED_EDGE('',*,*,#3762,.T.);
#5009=ORIENTED_EDGE('',*,*,#3763,.F.);
#5010=ORIENTED_EDGE('',*,*,#3764,.F.);
#5011=ORIENTED_EDGE('',*,*,#3765,.F.);
#5012=ORIENTED_EDGE('',*,*,#3766,.T.);
#5013=ORIENTED_EDGE('',*,*,#3767,.F.);
#5014=ORIENTED_EDGE('',*,*,#3736,.T.);
#5015=ORIENTED_EDGE('',*,*,#3768,.F.);
#5016=ORIENTED_EDGE('',*,*,#3738,.T.);
#5017=ORIENTED_EDGE('',*,*,#3769,.F.);
#5018=ORIENTED_EDGE('',*,*,#3742,.F.);
#5019=ORIENTED_EDGE('',*,*,#3770,.F.);
#5020=ORIENTED_EDGE('',*,*,#3756,.F.);
#5021=ORIENTED_EDGE('',*,*,#3771,.F.);
#5022=ORIENTED_EDGE('',*,*,#3762,.F.);
#5023=ORIENTED_EDGE('',*,*,#3772,.F.);
#5024=ORIENTED_EDGE('',*,*,#3744,.F.);
#5025=ORIENTED_EDGE('',*,*,#3773,.F.);
#5026=ORIENTED_EDGE('',*,*,#3766,.F.);
#5027=ORIENTED_EDGE('',*,*,#3774,.F.);
#5028=ORIENTED_EDGE('',*,*,#3748,.F.);
#5029=ORIENTED_EDGE('',*,*,#3775,.F.);
#5030=ORIENTED_EDGE('',*,*,#3776,.F.);
#5031=ORIENTED_EDGE('',*,*,#3777,.F.);
#5032=ORIENTED_EDGE('',*,*,#3752,.F.);
#5033=ORIENTED_EDGE('',*,*,#3778,.F.);
#5034=ORIENTED_EDGE('',*,*,#3779,.F.);
#5035=ORIENTED_EDGE('',*,*,#3780,.F.);
#5036=ORIENTED_EDGE('',*,*,#3776,.T.);
#5037=ORIENTED_EDGE('',*,*,#3781,.T.);
#5038=ORIENTED_EDGE('',*,*,#3782,.F.);
#5039=ORIENTED_EDGE('',*,*,#3783,.F.);
#5040=ORIENTED_EDGE('',*,*,#3784,.F.);
#5041=ORIENTED_EDGE('',*,*,#3785,.F.);
#5042=ORIENTED_EDGE('',*,*,#3786,.F.);
#5043=ORIENTED_EDGE('',*,*,#3753,.T.);
#5044=ORIENTED_EDGE('',*,*,#3777,.T.);
#5045=ORIENTED_EDGE('',*,*,#3780,.T.);
#5046=ORIENTED_EDGE('',*,*,#3787,.T.);
#5047=ORIENTED_EDGE('',*,*,#3788,.F.);
#5048=ORIENTED_EDGE('',*,*,#3789,.F.);
#5049=ORIENTED_EDGE('',*,*,#3790,.F.);
#5050=ORIENTED_EDGE('',*,*,#3791,.F.);
#5051=ORIENTED_EDGE('',*,*,#3792,.F.);
#5052=ORIENTED_EDGE('',*,*,#3793,.T.);
#5053=ORIENTED_EDGE('',*,*,#3749,.T.);
#5054=ORIENTED_EDGE('',*,*,#3774,.T.);
#5055=ORIENTED_EDGE('',*,*,#3765,.T.);
#5056=ORIENTED_EDGE('',*,*,#3794,.T.);
#5057=ORIENTED_EDGE('',*,*,#3795,.F.);
#5058=ORIENTED_EDGE('',*,*,#3796,.F.);
#5059=ORIENTED_EDGE('',*,*,#3797,.F.);
#5060=ORIENTED_EDGE('',*,*,#3798,.F.);
#5061=ORIENTED_EDGE('',*,*,#3799,.F.);
#5062=ORIENTED_EDGE('',*,*,#3800,.T.);
#5063=ORIENTED_EDGE('',*,*,#3745,.T.);
#5064=ORIENTED_EDGE('',*,*,#3772,.T.);
#5065=ORIENTED_EDGE('',*,*,#3761,.T.);
#5066=ORIENTED_EDGE('',*,*,#3801,.T.);
#5067=ORIENTED_EDGE('',*,*,#3802,.F.);
#5068=ORIENTED_EDGE('',*,*,#3803,.F.);
#5069=ORIENTED_EDGE('',*,*,#3804,.F.);
#5070=ORIENTED_EDGE('',*,*,#3805,.F.);
#5071=ORIENTED_EDGE('',*,*,#3806,.F.);
#5072=ORIENTED_EDGE('',*,*,#3807,.T.);
#5073=ORIENTED_EDGE('',*,*,#3739,.T.);
#5074=ORIENTED_EDGE('',*,*,#3769,.T.);
#5075=ORIENTED_EDGE('',*,*,#3755,.T.);
#5076=ORIENTED_EDGE('',*,*,#3808,.F.);
#5077=ORIENTED_EDGE('',*,*,#3809,.T.);
#5078=ORIENTED_EDGE('',*,*,#3810,.T.);
#5079=ORIENTED_EDGE('',*,*,#3811,.T.);
#5080=ORIENTED_EDGE('',*,*,#3812,.F.);
#5081=ORIENTED_EDGE('',*,*,#3754,.T.);
#5082=ORIENTED_EDGE('',*,*,#3793,.F.);
#5083=ORIENTED_EDGE('',*,*,#3813,.T.);
#5084=ORIENTED_EDGE('',*,*,#3781,.F.);
#5085=ORIENTED_EDGE('',*,*,#3814,.T.);
#5086=ORIENTED_EDGE('',*,*,#3787,.F.);
#5087=ORIENTED_EDGE('',*,*,#3779,.T.);
#5088=ORIENTED_EDGE('',*,*,#3815,.F.);
#5089=ORIENTED_EDGE('',*,*,#3816,.T.);
#5090=ORIENTED_EDGE('',*,*,#3794,.F.);
#5091=ORIENTED_EDGE('',*,*,#3764,.T.);
#5092=ORIENTED_EDGE('',*,*,#3817,.F.);
#5093=ORIENTED_EDGE('',*,*,#3818,.T.);
#5094=ORIENTED_EDGE('',*,*,#3801,.F.);
#5095=ORIENTED_EDGE('',*,*,#3760,.T.);
#5096=ORIENTED_EDGE('',*,*,#3819,.F.);
#5097=ORIENTED_EDGE('',*,*,#3820,.T.);
#5098=ORIENTED_EDGE('',*,*,#3821,.T.);
#5099=ORIENTED_EDGE('',*,*,#3808,.T.);
#5100=ORIENTED_EDGE('',*,*,#3758,.T.);
#5101=ORIENTED_EDGE('',*,*,#3822,.T.);
#5102=ORIENTED_EDGE('',*,*,#3823,.F.);
#5103=ORIENTED_EDGE('',*,*,#3824,.T.);
#5104=ORIENTED_EDGE('',*,*,#3825,.F.);
#5105=ORIENTED_EDGE('',*,*,#3826,.T.);
#5106=ORIENTED_EDGE('',*,*,#3827,.F.);
#5107=ORIENTED_EDGE('',*,*,#3828,.T.);
#5108=ORIENTED_EDGE('',*,*,#3829,.F.);
#5109=ORIENTED_EDGE('',*,*,#3830,.T.);
#5110=ORIENTED_EDGE('',*,*,#3740,.T.);
#5111=ORIENTED_EDGE('',*,*,#3812,.T.);
#5112=ORIENTED_EDGE('',*,*,#3831,.T.);
#5113=ORIENTED_EDGE('',*,*,#3832,.T.);
#5114=ORIENTED_EDGE('',*,*,#3833,.F.);
#5115=ORIENTED_EDGE('',*,*,#3746,.T.);
#5116=ORIENTED_EDGE('',*,*,#3807,.F.);
#5117=ORIENTED_EDGE('',*,*,#3834,.T.);
#5118=ORIENTED_EDGE('',*,*,#3835,.F.);
#5119=ORIENTED_EDGE('',*,*,#3750,.T.);
#5120=ORIENTED_EDGE('',*,*,#3800,.F.);
#5121=ORIENTED_EDGE('',*,*,#3836,.T.);
#5122=ORIENTED_EDGE('',*,*,#3837,.F.);
#5123=ORIENTED_EDGE('',*,*,#3838,.T.);
#5124=ORIENTED_EDGE('',*,*,#3839,.T.);
#5125=ORIENTED_EDGE('',*,*,#3840,.T.);
#5126=ORIENTED_EDGE('',*,*,#3841,.T.);
#5127=ORIENTED_EDGE('',*,*,#3842,.T.);
#5128=ORIENTED_EDGE('',*,*,#3843,.F.);
#5129=ORIENTED_EDGE('',*,*,#3844,.F.);
#5130=ORIENTED_EDGE('',*,*,#3845,.T.);
#5131=ORIENTED_EDGE('',*,*,#3768,.T.);
#5132=ORIENTED_EDGE('',*,*,#3845,.F.);
#5133=ORIENTED_EDGE('',*,*,#3846,.F.);
#5134=ORIENTED_EDGE('',*,*,#3847,.T.);
#5135=ORIENTED_EDGE('',*,*,#3767,.T.);
#5136=ORIENTED_EDGE('',*,*,#3847,.F.);
#5137=ORIENTED_EDGE('',*,*,#3848,.F.);
#5138=ORIENTED_EDGE('',*,*,#3843,.T.);
#5139=ORIENTED_EDGE('',*,*,#3849,.F.);
#5140=ORIENTED_EDGE('',*,*,#3850,.F.);
#5141=ORIENTED_EDGE('',*,*,#3851,.F.);
#5142=ORIENTED_EDGE('',*,*,#3852,.F.);
#5143=ORIENTED_EDGE('',*,*,#3782,.T.);
#5144=ORIENTED_EDGE('',*,*,#3813,.F.);
#5145=ORIENTED_EDGE('',*,*,#3792,.T.);
#5146=ORIENTED_EDGE('',*,*,#3853,.T.);
#5147=ORIENTED_EDGE('',*,*,#3848,.T.);
#5148=ORIENTED_EDGE('',*,*,#3854,.T.);
#5149=ORIENTED_EDGE('',*,*,#3855,.T.);
#5150=ORIENTED_EDGE('',*,*,#3838,.F.);
#5151=ORIENTED_EDGE('',*,*,#3783,.T.);
#5152=ORIENTED_EDGE('',*,*,#3853,.F.);
#5153=ORIENTED_EDGE('',*,*,#3791,.T.);
#5154=ORIENTED_EDGE('',*,*,#3856,.F.);
#5155=ORIENTED_EDGE('',*,*,#3852,.T.);
#5156=ORIENTED_EDGE('',*,*,#3857,.F.);
#5157=ORIENTED_EDGE('',*,*,#3858,.F.);
#5158=ORIENTED_EDGE('',*,*,#3854,.F.);
#5159=ORIENTED_EDGE('',*,*,#3784,.T.);
#5160=ORIENTED_EDGE('',*,*,#3856,.T.);
#5161=ORIENTED_EDGE('',*,*,#3790,.T.);
#5162=ORIENTED_EDGE('',*,*,#3859,.T.);
#5163=ORIENTED_EDGE('',*,*,#3717,.T.);
#5164=ORIENTED_EDGE('',*,*,#3726,.T.);
#5165=ORIENTED_EDGE('',*,*,#3844,.T.);
#5166=ORIENTED_EDGE('',*,*,#3851,.T.);
#5167=ORIENTED_EDGE('',*,*,#3860,.T.);
#5168=ORIENTED_EDGE('',*,*,#3861,.T.);
#5169=ORIENTED_EDGE('',*,*,#3857,.T.);
#5170=ORIENTED_EDGE('',*,*,#3785,.T.);
#5171=ORIENTED_EDGE('',*,*,#3859,.F.);
#5172=ORIENTED_EDGE('',*,*,#3789,.T.);
#5173=ORIENTED_EDGE('',*,*,#3862,.F.);
#5174=ORIENTED_EDGE('',*,*,#3786,.T.);
#5175=ORIENTED_EDGE('',*,*,#3862,.T.);
#5176=ORIENTED_EDGE('',*,*,#3788,.T.);
#5177=ORIENTED_EDGE('',*,*,#3814,.F.);
#5178=ORIENTED_EDGE('',*,*,#3849,.T.);
#5179=ORIENTED_EDGE('',*,*,#3842,.F.);
#5180=ORIENTED_EDGE('',*,*,#3863,.T.);
#5181=ORIENTED_EDGE('',*,*,#3864,.T.);
#5182=ORIENTED_EDGE('',*,*,#3751,.T.);
#5183=ORIENTED_EDGE('',*,*,#3837,.T.);
#5184=ORIENTED_EDGE('',*,*,#3865,.F.);
#5185=ORIENTED_EDGE('',*,*,#3866,.F.);
#5186=ORIENTED_EDGE('',*,*,#3867,.F.);
#5187=ORIENTED_EDGE('',*,*,#3868,.F.);
#5188=ORIENTED_EDGE('',*,*,#3869,.F.);
#5189=ORIENTED_EDGE('',*,*,#3815,.T.);
#5190=ORIENTED_EDGE('',*,*,#3778,.T.);
#5191=ORIENTED_EDGE('',*,*,#3775,.T.);
#5192=ORIENTED_EDGE('',*,*,#3865,.T.);
#5193=ORIENTED_EDGE('',*,*,#3836,.F.);
#5194=ORIENTED_EDGE('',*,*,#3799,.T.);
#5195=ORIENTED_EDGE('',*,*,#3870,.T.);
#5196=ORIENTED_EDGE('',*,*,#3866,.T.);
#5197=ORIENTED_EDGE('',*,*,#3870,.F.);
#5198=ORIENTED_EDGE('',*,*,#3798,.T.);
#5199=ORIENTED_EDGE('',*,*,#3871,.F.);
#5200=ORIENTED_EDGE('',*,*,#3867,.T.);
#5201=ORIENTED_EDGE('',*,*,#3871,.T.);
#5202=ORIENTED_EDGE('',*,*,#3797,.T.);
#5203=ORIENTED_EDGE('',*,*,#3872,.T.);
#5204=ORIENTED_EDGE('',*,*,#3868,.T.);
#5205=ORIENTED_EDGE('',*,*,#3872,.F.);
#5206=ORIENTED_EDGE('',*,*,#3796,.T.);
#5207=ORIENTED_EDGE('',*,*,#3873,.F.);
#5208=ORIENTED_EDGE('',*,*,#3869,.T.);
#5209=ORIENTED_EDGE('',*,*,#3873,.T.);
#5210=ORIENTED_EDGE('',*,*,#3795,.T.);
#5211=ORIENTED_EDGE('',*,*,#3816,.F.);
#5212=ORIENTED_EDGE('',*,*,#3747,.T.);
#5213=ORIENTED_EDGE('',*,*,#3835,.T.);
#5214=ORIENTED_EDGE('',*,*,#3874,.F.);
#5215=ORIENTED_EDGE('',*,*,#3875,.F.);
#5216=ORIENTED_EDGE('',*,*,#3876,.F.);
#5217=ORIENTED_EDGE('',*,*,#3877,.F.);
#5218=ORIENTED_EDGE('',*,*,#3878,.F.);
#5219=ORIENTED_EDGE('',*,*,#3817,.T.);
#5220=ORIENTED_EDGE('',*,*,#3763,.T.);
#5221=ORIENTED_EDGE('',*,*,#3773,.T.);
#5222=ORIENTED_EDGE('',*,*,#3874,.T.);
#5223=ORIENTED_EDGE('',*,*,#3834,.F.);
#5224=ORIENTED_EDGE('',*,*,#3806,.T.);
#5225=ORIENTED_EDGE('',*,*,#3879,.T.);
#5226=ORIENTED_EDGE('',*,*,#3875,.T.);
#5227=ORIENTED_EDGE('',*,*,#3879,.F.);
#5228=ORIENTED_EDGE('',*,*,#3805,.T.);
#5229=ORIENTED_EDGE('',*,*,#3880,.F.);
#5230=ORIENTED_EDGE('',*,*,#3876,.T.);
#5231=ORIENTED_EDGE('',*,*,#3880,.T.);
#5232=ORIENTED_EDGE('',*,*,#3804,.T.);
#5233=ORIENTED_EDGE('',*,*,#3881,.T.);
#5234=ORIENTED_EDGE('',*,*,#3720,.T.);
#5235=ORIENTED_EDGE('',*,*,#3723,.T.);
#5236=ORIENTED_EDGE('',*,*,#3846,.T.);
#5237=ORIENTED_EDGE('',*,*,#3877,.T.);
#5238=ORIENTED_EDGE('',*,*,#3881,.F.);
#5239=ORIENTED_EDGE('',*,*,#3803,.T.);
#5240=ORIENTED_EDGE('',*,*,#3882,.F.);
#5241=ORIENTED_EDGE('',*,*,#3878,.T.);
#5242=ORIENTED_EDGE('',*,*,#3882,.T.);
#5243=ORIENTED_EDGE('',*,*,#3802,.T.);
#5244=ORIENTED_EDGE('',*,*,#3818,.F.);
#5245=ORIENTED_EDGE('',*,*,#3743,.T.);
#5246=ORIENTED_EDGE('',*,*,#3833,.T.);
#5247=ORIENTED_EDGE('',*,*,#3883,.F.);
#5248=ORIENTED_EDGE('',*,*,#3884,.F.);
#5249=ORIENTED_EDGE('',*,*,#3885,.F.);
#5250=ORIENTED_EDGE('',*,*,#3886,.F.);
#5251=ORIENTED_EDGE('',*,*,#3887,.F.);
#5252=ORIENTED_EDGE('',*,*,#3819,.T.);
#5253=ORIENTED_EDGE('',*,*,#3759,.T.);
#5254=ORIENTED_EDGE('',*,*,#3771,.T.);
#5255=ORIENTED_EDGE('',*,*,#3883,.T.);
#5256=ORIENTED_EDGE('',*,*,#3832,.F.);
#5257=ORIENTED_EDGE('',*,*,#3888,.T.);
#5258=ORIENTED_EDGE('',*,*,#3889,.T.);
#5259=ORIENTED_EDGE('',*,*,#3884,.T.);
#5260=ORIENTED_EDGE('',*,*,#3889,.F.);
#5261=ORIENTED_EDGE('',*,*,#3890,.F.);
#5262=ORIENTED_EDGE('',*,*,#3891,.F.);
#5263=ORIENTED_EDGE('',*,*,#3885,.T.);
#5264=ORIENTED_EDGE('',*,*,#3891,.T.);
#5265=ORIENTED_EDGE('',*,*,#3892,.T.);
#5266=ORIENTED_EDGE('',*,*,#3893,.T.);
#5267=ORIENTED_EDGE('',*,*,#3887,.T.);
#5268=ORIENTED_EDGE('',*,*,#3894,.T.);
#5269=ORIENTED_EDGE('',*,*,#3895,.T.);
#5270=ORIENTED_EDGE('',*,*,#3820,.F.);
#5271=ORIENTED_EDGE('',*,*,#3886,.T.);
#5272=ORIENTED_EDGE('',*,*,#3893,.F.);
#5273=ORIENTED_EDGE('',*,*,#3896,.F.);
#5274=ORIENTED_EDGE('',*,*,#3894,.F.);
#5275=ORIENTED_EDGE('',*,*,#3897,.T.);
#5276=ORIENTED_EDGE('',*,*,#3898,.T.);
#5277=ORIENTED_EDGE('',*,*,#3896,.T.);
#5278=ORIENTED_EDGE('',*,*,#3899,.T.);
#5279=ORIENTED_EDGE('',*,*,#3900,.T.);
#5280=ORIENTED_EDGE('',*,*,#3901,.T.);
#5281=ORIENTED_EDGE('',*,*,#3890,.T.);
#5282=ORIENTED_EDGE('',*,*,#3902,.T.);
#5283=ORIENTED_EDGE('',*,*,#3903,.T.);
#5284=ORIENTED_EDGE('',*,*,#3897,.F.);
#5285=ORIENTED_EDGE('',*,*,#3892,.F.);
#5286=ORIENTED_EDGE('',*,*,#3903,.F.);
#5287=ORIENTED_EDGE('',*,*,#3810,.F.);
#5288=ORIENTED_EDGE('',*,*,#3831,.F.);
#5289=ORIENTED_EDGE('',*,*,#3811,.F.);
#5290=ORIENTED_EDGE('',*,*,#3902,.F.);
#5291=ORIENTED_EDGE('',*,*,#3888,.F.);
#5292=ORIENTED_EDGE('',*,*,#3904,.T.);
#5293=ORIENTED_EDGE('',*,*,#3858,.T.);
#5294=ORIENTED_EDGE('',*,*,#3905,.T.);
#5295=ORIENTED_EDGE('',*,*,#3905,.F.);
#5296=ORIENTED_EDGE('',*,*,#3861,.F.);
#5297=ORIENTED_EDGE('',*,*,#3901,.F.);
#5298=ORIENTED_EDGE('',*,*,#3906,.F.);
#5299=ORIENTED_EDGE('',*,*,#3839,.F.);
#5300=ORIENTED_EDGE('',*,*,#3855,.F.);
#5301=ORIENTED_EDGE('',*,*,#3904,.F.);
#5302=ORIENTED_EDGE('',*,*,#3907,.F.);
#5303=ORIENTED_EDGE('',*,*,#3841,.F.);
#5304=ORIENTED_EDGE('',*,*,#3908,.F.);
#5305=ORIENTED_EDGE('',*,*,#3900,.F.);
#5306=ORIENTED_EDGE('',*,*,#3863,.F.);
#5307=ORIENTED_EDGE('',*,*,#3850,.T.);
#5308=ORIENTED_EDGE('',*,*,#3864,.F.);
#5309=ORIENTED_EDGE('',*,*,#3899,.F.);
#5310=ORIENTED_EDGE('',*,*,#3860,.F.);
#5311=ORIENTED_EDGE('',*,*,#3821,.F.);
#5312=ORIENTED_EDGE('',*,*,#3895,.F.);
#5313=ORIENTED_EDGE('',*,*,#3898,.F.);
#5314=ORIENTED_EDGE('',*,*,#3809,.F.);
#5315=ORIENTED_EDGE('',*,*,#3907,.T.);
#5316=ORIENTED_EDGE('',*,*,#3906,.T.);
#5317=ORIENTED_EDGE('',*,*,#3908,.T.);
#5318=ORIENTED_EDGE('',*,*,#3840,.F.);
#5319=ORIENTED_EDGE('',*,*,#3909,.F.);
#5320=ORIENTED_EDGE('',*,*,#3910,.F.);
#5321=ORIENTED_EDGE('',*,*,#3911,.F.);
#5322=ORIENTED_EDGE('',*,*,#3912,.F.);
#5323=ORIENTED_EDGE('',*,*,#3913,.F.);
#5324=ORIENTED_EDGE('',*,*,#3914,.F.);
#5325=ORIENTED_EDGE('',*,*,#3915,.F.);
#5326=ORIENTED_EDGE('',*,*,#3916,.F.);
#5327=ORIENTED_EDGE('',*,*,#3917,.F.);
#5328=ORIENTED_EDGE('',*,*,#3909,.T.);
#5329=ORIENTED_EDGE('',*,*,#3918,.T.);
#5330=ORIENTED_EDGE('',*,*,#3916,.T.);
#5331=ORIENTED_EDGE('',*,*,#3919,.T.);
#5332=ORIENTED_EDGE('',*,*,#3829,.T.);
#5333=ORIENTED_EDGE('',*,*,#3920,.T.);
#5334=ORIENTED_EDGE('',*,*,#3917,.T.);
#5335=ORIENTED_EDGE('',*,*,#3921,.T.);
#5336=ORIENTED_EDGE('',*,*,#3922,.F.);
#5337=ORIENTED_EDGE('',*,*,#3923,.F.);
#5338=ORIENTED_EDGE('',*,*,#3924,.F.);
#5339=ORIENTED_EDGE('',*,*,#3923,.T.);
#5340=ORIENTED_EDGE('',*,*,#3925,.T.);
#5341=ORIENTED_EDGE('',*,*,#3913,.T.);
#5342=ORIENTED_EDGE('',*,*,#3926,.T.);
#5343=ORIENTED_EDGE('',*,*,#3915,.T.);
#5344=ORIENTED_EDGE('',*,*,#3927,.T.);
#5345=ORIENTED_EDGE('',*,*,#3924,.T.);
#5346=ORIENTED_EDGE('',*,*,#3928,.T.);
#5347=ORIENTED_EDGE('',*,*,#3827,.T.);
#5348=ORIENTED_EDGE('',*,*,#3929,.T.);
#5349=ORIENTED_EDGE('',*,*,#3922,.T.);
#5350=ORIENTED_EDGE('',*,*,#3930,.T.);
#5351=ORIENTED_EDGE('',*,*,#3825,.T.);
#5352=ORIENTED_EDGE('',*,*,#3931,.T.);
#5353=ORIENTED_EDGE('',*,*,#3914,.T.);
#5354=ORIENTED_EDGE('',*,*,#3932,.T.);
#5355=ORIENTED_EDGE('',*,*,#3912,.T.);
#5356=ORIENTED_EDGE('',*,*,#3933,.T.);
#5357=ORIENTED_EDGE('',*,*,#3910,.T.);
#5358=ORIENTED_EDGE('',*,*,#3934,.T.);
#5359=ORIENTED_EDGE('',*,*,#3823,.T.);
#5360=ORIENTED_EDGE('',*,*,#3935,.T.);
#5361=ORIENTED_EDGE('',*,*,#3911,.T.);
#5362=ORIENTED_EDGE('',*,*,#3936,.T.);
#5363=ORIENTED_EDGE('',*,*,#3930,.F.);
#5364=ORIENTED_EDGE('',*,*,#3927,.F.);
#5365=ORIENTED_EDGE('',*,*,#3920,.F.);
#5366=ORIENTED_EDGE('',*,*,#3828,.F.);
#5367=ORIENTED_EDGE('',*,*,#3741,.T.);
#5368=ORIENTED_EDGE('',*,*,#3830,.F.);
#5369=ORIENTED_EDGE('',*,*,#3921,.F.);
#5370=ORIENTED_EDGE('',*,*,#3918,.F.);
#5371=ORIENTED_EDGE('',*,*,#3935,.F.);
#5372=ORIENTED_EDGE('',*,*,#3822,.F.);
#5373=ORIENTED_EDGE('',*,*,#3757,.T.);
#5374=ORIENTED_EDGE('',*,*,#3770,.T.);
#5375=ORIENTED_EDGE('',*,*,#3926,.F.);
#5376=ORIENTED_EDGE('',*,*,#3934,.F.);
#5377=ORIENTED_EDGE('',*,*,#3919,.F.);
#5378=ORIENTED_EDGE('',*,*,#3928,.F.);
#5379=ORIENTED_EDGE('',*,*,#3731,.T.);
#5380=ORIENTED_EDGE('',*,*,#3727,.T.);
#5381=ORIENTED_EDGE('',*,*,#3724,.T.);
#5382=ORIENTED_EDGE('',*,*,#3721,.T.);
#5383=ORIENTED_EDGE('',*,*,#3718,.T.);
#5384=ORIENTED_EDGE('',*,*,#3715,.T.);
#5385=ORIENTED_EDGE('',*,*,#3931,.F.);
#5386=ORIENTED_EDGE('',*,*,#3824,.F.);
#5387=ORIENTED_EDGE('',*,*,#3936,.F.);
#5388=ORIENTED_EDGE('',*,*,#3933,.F.);
#5389=ORIENTED_EDGE('',*,*,#3929,.F.);
#5390=ORIENTED_EDGE('',*,*,#3826,.F.);
#5391=ORIENTED_EDGE('',*,*,#3932,.F.);
#5392=ORIENTED_EDGE('',*,*,#3925,.F.);
#6627=CYLINDRICAL_SURFACE('',#7424,0.15);
#6628=CYLINDRICAL_SURFACE('',#7427,0.15);
#6629=CYLINDRICAL_SURFACE('',#7430,0.15);
#6630=CYLINDRICAL_SURFACE('',#7433,0.15);
#6631=CYLINDRICAL_SURFACE('',#7436,0.3);
#6632=CYLINDRICAL_SURFACE('',#7441,0.3);
#6633=CYLINDRICAL_SURFACE('',#7446,0.17);
#6634=CYLINDRICAL_SURFACE('',#7448,0.17);
#6635=CYLINDRICAL_SURFACE('',#7472,0.4);
#6636=CYLINDRICAL_SURFACE('',#7474,0.4);
#6637=CYLINDRICAL_SURFACE('',#7498,0.1);
#6638=CYLINDRICAL_SURFACE('',#7502,0.1);
#6639=CYLINDRICAL_SURFACE('',#7516,0.3);
#6640=CYLINDRICAL_SURFACE('',#7521,0.3);
#6825=ADVANCED_FACE('',(#903),#6627,.F.);
#6826=ADVANCED_FACE('',(#904),#6628,.F.);
#6827=ADVANCED_FACE('',(#905),#6629,.F.);
#6828=ADVANCED_FACE('',(#906),#6630,.F.);
#6829=ADVANCED_FACE('',(#907),#6631,.F.);
#6830=ADVANCED_FACE('',(#908,#601),#706,.F.);
#6831=ADVANCED_FACE('',(#909),#6632,.F.);
#6832=ADVANCED_FACE('',(#910,#602),#707,.F.);
#6833=ADVANCED_FACE('',(#911),#6633,.F.);
#6834=ADVANCED_FACE('',(#912),#6634,.F.);
#6835=ADVANCED_FACE('',(#913),#708,.F.);
#6836=ADVANCED_FACE('',(#914),#709,.F.);
#6837=ADVANCED_FACE('',(#915),#710,.F.);
#6838=ADVANCED_FACE('',(#916),#711,.F.);
#6839=ADVANCED_FACE('',(#917),#712,.F.);
#6840=ADVANCED_FACE('',(#918),#713,.F.);
#6841=ADVANCED_FACE('',(#919),#714,.F.);
#6842=ADVANCED_FACE('',(#920,#603),#715,.F.);
#6843=ADVANCED_FACE('',(#921,#604),#716,.F.);
#6844=ADVANCED_FACE('',(#922),#717,.F.);
#6845=ADVANCED_FACE('',(#923),#718,.F.);
#6846=ADVANCED_FACE('',(#924),#719,.F.);
#6847=ADVANCED_FACE('',(#925),#720,.F.);
#6848=ADVANCED_FACE('',(#926),#721,.F.);
#6849=ADVANCED_FACE('',(#927),#722,.T.);
#6850=ADVANCED_FACE('',(#928),#723,.T.);
#6851=ADVANCED_FACE('',(#929),#724,.T.);
#6852=ADVANCED_FACE('',(#930),#725,.T.);
#6853=ADVANCED_FACE('',(#931),#726,.T.);
#6854=ADVANCED_FACE('',(#932,#605),#727,.F.);
#6855=ADVANCED_FACE('',(#933),#6635,.T.);
#6856=ADVANCED_FACE('',(#934),#6636,.T.);
#6857=ADVANCED_FACE('',(#935),#728,.T.);
#6858=ADVANCED_FACE('',(#936),#92,.T.);
#6859=ADVANCED_FACE('',(#937),#93,.T.);
#6860=ADVANCED_FACE('',(#938),#94,.T.);
#6861=ADVANCED_FACE('',(#939),#95,.T.);
#6862=ADVANCED_FACE('',(#940,#606,#607,#608),#729,.F.);
#6863=ADVANCED_FACE('',(#941),#730,.F.);
#6864=ADVANCED_FACE('',(#942),#96,.T.);
#6865=ADVANCED_FACE('',(#943),#97,.T.);
#6866=ADVANCED_FACE('',(#944),#98,.T.);
#6867=ADVANCED_FACE('',(#945),#731,.T.);
#6868=ADVANCED_FACE('',(#946),#99,.T.);
#6869=ADVANCED_FACE('',(#947),#100,.T.);
#6870=ADVANCED_FACE('',(#948),#732,.F.);
#6871=ADVANCED_FACE('',(#949),#101,.T.);
#6872=ADVANCED_FACE('',(#950),#102,.T.);
#6873=ADVANCED_FACE('',(#951),#733,.T.);
#6874=ADVANCED_FACE('',(#952),#103,.T.);
#6875=ADVANCED_FACE('',(#953),#104,.T.);
#6876=ADVANCED_FACE('',(#954,#609,#610,#611),#734,.F.);
#6877=ADVANCED_FACE('',(#955),#105,.T.);
#6878=ADVANCED_FACE('',(#956),#106,.T.);
#6879=ADVANCED_FACE('',(#957),#735,.T.);
#6880=ADVANCED_FACE('',(#958),#107,.T.);
#6881=ADVANCED_FACE('',(#959),#108,.T.);
#6882=ADVANCED_FACE('',(#960),#736,.F.);
#6883=ADVANCED_FACE('',(#961),#109,.T.);
#6884=ADVANCED_FACE('',(#962),#110,.T.);
#6885=ADVANCED_FACE('',(#963),#76,.F.);
#6886=ADVANCED_FACE('',(#964),#77,.F.);
#6887=ADVANCED_FACE('',(#965),#78,.F.);
#6888=ADVANCED_FACE('',(#966),#6637,.F.);
#6889=ADVANCED_FACE('',(#967),#111,.T.);
#6890=ADVANCED_FACE('',(#968),#79,.F.);
#6891=ADVANCED_FACE('',(#969),#6638,.F.);
#6892=ADVANCED_FACE('',(#970),#112,.T.);
#6893=ADVANCED_FACE('',(#971),#113,.T.);
#6894=ADVANCED_FACE('',(#972),#114,.T.);
#6895=ADVANCED_FACE('',(#973),#115,.T.);
#6896=ADVANCED_FACE('',(#974),#737,.T.);
#6897=ADVANCED_FACE('',(#975),#80,.T.);
#6898=ADVANCED_FACE('',(#976),#81,.T.);
#6899=ADVANCED_FACE('',(#977),#82,.T.);
#6900=ADVANCED_FACE('',(#978),#6639,.T.);
#6901=ADVANCED_FACE('',(#979),#116,.F.);
#6902=ADVANCED_FACE('',(#980),#83,.T.);
#6903=ADVANCED_FACE('',(#981),#6640,.T.);
#6904=ADVANCED_FACE('',(#982),#117,.F.);
#6905=ADVANCED_FACE('',(#983),#118,.F.);
#6906=ADVANCED_FACE('',(#984),#119,.F.);
#6907=ADVANCED_FACE('',(#985),#120,.F.);
#6908=ADVANCED_FACE('',(#986),#121,.F.);
#6909=ADVANCED_FACE('',(#987),#122,.F.);
#6910=ADVANCED_FACE('',(#988),#738,.F.);
#6911=ADVANCED_FACE('',(#989,#612,#613,#614,#615,#616,#617),#739,.T.);
#6912=ADVANCED_FACE('',(#990),#123,.F.);
#6913=ADVANCED_FACE('',(#991),#740,.F.);
#7155=CLOSED_SHELL('',(#6825,#6826,#6827,#6828,#6829,#6830,#6831,#6832,
#6833,#6834,#6835,#6836,#6837,#6838,#6839,#6840,#6841,#6842,#6843,#6844,
#6845,#6846,#6847,#6848,#6849,#6850,#6851,#6852,#6853,#6854,#6855,#6856,
#6857,#6858,#6859,#6860,#6861,#6862,#6863,#6864,#6865,#6866,#6867,#6868,
#6869,#6870,#6871,#6872,#6873,#6874,#6875,#6876,#6877,#6878,#6879,#6880,
#6881,#6882,#6883,#6884,#6885,#6886,#6887,#6888,#6889,#6890,#6891,#6892,
#6893,#6894,#6895,#6896,#6897,#6898,#6899,#6900,#6901,#6902,#6903,#6904,
#6905,#6906,#6907,#6908,#6909,#6910,#6911,#6912,#6913));
#7423=AXIS2_PLACEMENT_3D('',#9812,#8263,#8264);
#7424=AXIS2_PLACEMENT_3D('',#9813,#8265,#8266);
#7425=AXIS2_PLACEMENT_3D('',#9815,#8267,#8268);
#7426=AXIS2_PLACEMENT_3D('',#9818,#8270,#8271);
#7427=AXIS2_PLACEMENT_3D('',#9819,#8272,#8273);
#7428=AXIS2_PLACEMENT_3D('',#9821,#8274,#8275);
#7429=AXIS2_PLACEMENT_3D('',#9824,#8277,#8278);
#7430=AXIS2_PLACEMENT_3D('',#9825,#8279,#8280);
#7431=AXIS2_PLACEMENT_3D('',#9827,#8281,#8282);
#7432=AXIS2_PLACEMENT_3D('',#9830,#8284,#8285);
#7433=AXIS2_PLACEMENT_3D('',#9831,#8286,#8287);
#7434=AXIS2_PLACEMENT_3D('',#9833,#8288,#8289);
#7435=AXIS2_PLACEMENT_3D('',#9836,#8291,#8292);
#7436=AXIS2_PLACEMENT_3D('',#9837,#8293,#8294);
#7437=AXIS2_PLACEMENT_3D('',#9839,#8295,#8296);
#7438=AXIS2_PLACEMENT_3D('',#9842,#8298,#8299);
#7439=AXIS2_PLACEMENT_3D('',#9843,#8300,#8301);
#7440=AXIS2_PLACEMENT_3D('',#9845,#8302,#8303);
#7441=AXIS2_PLACEMENT_3D('',#9846,#8304,#8305);
#7442=AXIS2_PLACEMENT_3D('',#9848,#8306,#8307);
#7443=AXIS2_PLACEMENT_3D('',#9851,#8309,#8310);
#7444=AXIS2_PLACEMENT_3D('',#9852,#8311,#8312);
#7445=AXIS2_PLACEMENT_3D('',#9854,#8313,#8314);
#7446=AXIS2_PLACEMENT_3D('',#9855,#8315,#8316);
#7447=AXIS2_PLACEMENT_3D('',#9858,#8318,#8319);
#7448=AXIS2_PLACEMENT_3D('',#9859,#8320,#8321);
#7449=AXIS2_PLACEMENT_3D('',#9862,#8323,#8324);
#7450=AXIS2_PLACEMENT_3D('',#9863,#8325,#8326);
#7451=AXIS2_PLACEMENT_3D('',#9872,#8331,#8332);
#7452=AXIS2_PLACEMENT_3D('',#9881,#8337,#8338);
#7453=AXIS2_PLACEMENT_3D('',#9890,#8343,#8344);
#7454=AXIS2_PLACEMENT_3D('',#9899,#8349,#8350);
#7455=AXIS2_PLACEMENT_3D('',#9908,#8355,#8356);
#7456=AXIS2_PLACEMENT_3D('',#9917,#8361,#8362);
#7457=AXIS2_PLACEMENT_3D('',#9926,#8367,#8368);
#7458=AXIS2_PLACEMENT_3D('',#9928,#8369,#8370);
#7459=AXIS2_PLACEMENT_3D('',#9929,#8371,#8372);
#7460=AXIS2_PLACEMENT_3D('',#9931,#8373,#8374);
#7461=AXIS2_PLACEMENT_3D('',#9932,#8375,#8376);
#7462=AXIS2_PLACEMENT_3D('',#9935,#8379,#8380);
#7463=AXIS2_PLACEMENT_3D('',#9938,#8383,#8384);
#7464=AXIS2_PLACEMENT_3D('',#9941,#8387,#8388);
#7465=AXIS2_PLACEMENT_3D('',#9947,#8392,#8393);
#7466=AXIS2_PLACEMENT_3D('',#9953,#8397,#8398);
#7467=AXIS2_PLACEMENT_3D('',#10030,#8401,#8402);
#7468=AXIS2_PLACEMENT_3D('',#10108,#8406,#8407);
#7469=AXIS2_PLACEMENT_3D('',#10186,#8411,#8412);
#7470=AXIS2_PLACEMENT_3D('',#10264,#8416,#8417);
#7471=AXIS2_PLACEMENT_3D('',#10280,#8421,#8422);
#7472=AXIS2_PLACEMENT_3D('',#10604,#8434,#8435);
#7473=AXIS2_PLACEMENT_3D('',#10606,#8436,#8437);
#7474=AXIS2_PLACEMENT_3D('',#10608,#8439,#8440);
#7475=AXIS2_PLACEMENT_3D('',#10610,#8441,#8442);
#7476=AXIS2_PLACEMENT_3D('',#10612,#8444,#8445);
#7477=AXIS2_PLACEMENT_3D('',#10780,#8447,#8448);
#7478=AXIS2_PLACEMENT_3D('',#10781,#8449,#8450);
#7479=AXIS2_PLACEMENT_3D('',#10786,#8451,#8452);
#7480=AXIS2_PLACEMENT_3D('',#10858,#8454,#8455);
#7481=AXIS2_PLACEMENT_3D('',#10976,#8457,#8458);
#7482=AXIS2_PLACEMENT_3D('',#11021,#8459,#8460);
#7483=AXIS2_PLACEMENT_3D('',#11139,#8462,#8463);
#7484=AXIS2_PLACEMENT_3D('',#11184,#8464,#8465);
#7485=AXIS2_PLACEMENT_3D('',#11304,#8467,#8468);
#7486=AXIS2_PLACEMENT_3D('',#11309,#8469,#8470);
#7487=AXIS2_PLACEMENT_3D('',#11361,#8472,#8473);
#7488=AXIS2_PLACEMENT_3D('',#11362,#8474,#8475);
#7489=AXIS2_PLACEMENT_3D('',#11363,#8476,#8477);
#7490=AXIS2_PLACEMENT_3D('',#11364,#8478,#8479);
#7491=AXIS2_PLACEMENT_3D('',#11365,#8480,#8481);
#7492=AXIS2_PLACEMENT_3D('',#11366,#8482,#8483);
#7493=AXIS2_PLACEMENT_3D('',#11368,#8484,#8485);
#7494=AXIS2_PLACEMENT_3D('',#11369,#8486,#8487);
#7495=AXIS2_PLACEMENT_3D('',#11370,#8488,#8489);
#7496=AXIS2_PLACEMENT_3D('',#11371,#8490,#8491);
#7497=AXIS2_PLACEMENT_3D('',#11372,#8492,#8493);
#7498=AXIS2_PLACEMENT_3D('',#11373,#8494,#8495);
#7499=AXIS2_PLACEMENT_3D('',#11394,#8496,#8497);
#7500=AXIS2_PLACEMENT_3D('',#11396,#8498,#8499);
#7501=AXIS2_PLACEMENT_3D('',#11397,#8500,#8501);
#7502=AXIS2_PLACEMENT_3D('',#11398,#8502,#8503);
#7503=AXIS2_PLACEMENT_3D('',#11488,#8505,#8506);
#7504=AXIS2_PLACEMENT_3D('',#11489,#8507,#8508);
#7505=AXIS2_PLACEMENT_3D('',#11492,#8509,#8510);
#7506=AXIS2_PLACEMENT_3D('',#11494,#8511,#8512);
#7507=AXIS2_PLACEMENT_3D('',#11495,#8513,#8514);
#7508=AXIS2_PLACEMENT_3D('',#11496,#8515,#8516);
#7509=AXIS2_PLACEMENT_3D('',#11499,#8517,#8518);
#7510=AXIS2_PLACEMENT_3D('',#11501,#8519,#8520);
#7511=AXIS2_PLACEMENT_3D('',#11502,#8521,#8522);
#7512=AXIS2_PLACEMENT_3D('',#11503,#8523,#8524);
#7513=AXIS2_PLACEMENT_3D('',#11506,#8525,#8526);
#7514=AXIS2_PLACEMENT_3D('',#11508,#8527,#8528);
#7515=AXIS2_PLACEMENT_3D('',#11509,#8529,#8530);
#7516=AXIS2_PLACEMENT_3D('',#11510,#8531,#8532);
#7517=AXIS2_PLACEMENT_3D('',#11541,#8535,#8536);
#7518=AXIS2_PLACEMENT_3D('',#11544,#8537,#8538);
#7519=AXIS2_PLACEMENT_3D('',#11546,#8539,#8540);
#7520=AXIS2_PLACEMENT_3D('',#11547,#8541,#8542);
#7521=AXIS2_PLACEMENT_3D('',#11548,#8543,#8544);
#7522=AXIS2_PLACEMENT_3D('',#11728,#8547,#8548);
#7523=AXIS2_PLACEMENT_3D('',#11729,#8549,#8550);
#7524=AXIS2_PLACEMENT_3D('',#11746,#8551,#8552);
#8263=DIRECTION('axis',(0.,0.,1.));
#8264=DIRECTION('refdir',(1.,0.,0.));
#8265=DIRECTION('center_axis',(0.,0.,-1.));
#8266=DIRECTION('ref_axis',(1.,0.,0.));
#8267=DIRECTION('center_axis',(1.01338750660366E-31,-1.26069923670246E-19,
-1.));
#8268=DIRECTION('ref_axis',(1.,0.,0.));
#8269=DIRECTION('',(0.,0.,-1.));
#8270=DIRECTION('center_axis',(-1.01338750660366E-31,1.26069923670246E-19,
1.));
#8271=DIRECTION('ref_axis',(1.,0.,0.));
#8272=DIRECTION('center_axis',(0.,0.,-1.));
#8273=DIRECTION('ref_axis',(1.,0.,0.));
#8274=DIRECTION('center_axis',(1.01338750660366E-31,-1.26069923670246E-19,
-1.));
#8275=DIRECTION('ref_axis',(1.,0.,0.));
#8276=DIRECTION('',(0.,0.,-1.));
#8277=DIRECTION('center_axis',(-1.01338750660366E-31,1.26069923670246E-19,
1.));
#8278=DIRECTION('ref_axis',(1.,0.,0.));
#8279=DIRECTION('center_axis',(0.,0.,-1.));
#8280=DIRECTION('ref_axis',(1.,0.,0.));
#8281=DIRECTION('center_axis',(1.01338750660366E-31,-1.26069923670246E-19,
-1.));
#8282=DIRECTION('ref_axis',(1.,0.,0.));
#8283=DIRECTION('',(0.,0.,-1.));
#8284=DIRECTION('center_axis',(-1.01338750660366E-31,1.26069923670246E-19,
1.));
#8285=DIRECTION('ref_axis',(1.,0.,0.));
#8286=DIRECTION('center_axis',(0.,0.,-1.));
#8287=DIRECTION('ref_axis',(1.,0.,0.));
#8288=DIRECTION('center_axis',(1.01338750660366E-31,-1.26069923670246E-19,
-1.));
#8289=DIRECTION('ref_axis',(1.,0.,0.));
#8290=DIRECTION('',(0.,0.,-1.));
#8291=DIRECTION('center_axis',(-1.01338750660366E-31,1.26069923670246E-19,
1.));
#8292=DIRECTION('ref_axis',(1.,0.,0.));
#8293=DIRECTION('center_axis',(0.,0.,-1.));
#8294=DIRECTION('ref_axis',(1.,0.,0.));
#8295=DIRECTION('center_axis',(1.01338750660366E-31,-1.26069923670246E-19,
-1.));
#8296=DIRECTION('ref_axis',(1.,0.,0.));
#8297=DIRECTION('',(0.,0.,-1.));
#8298=DIRECTION('center_axis',(0.,0.,-1.));
#8299=DIRECTION('ref_axis',(1.,0.,0.));
#8300=DIRECTION('center_axis',(0.,0.,-1.));
#8301=DIRECTION('ref_axis',(1.,0.,0.));
#8302=DIRECTION('center_axis',(0.,0.,1.));
#8303=DIRECTION('ref_axis',(1.,0.,0.));
#8304=DIRECTION('center_axis',(0.,0.,-1.));
#8305=DIRECTION('ref_axis',(1.,0.,0.));
#8306=DIRECTION('center_axis',(1.01338750660366E-31,-1.26069923670246E-19,
-1.));
#8307=DIRECTION('ref_axis',(1.,0.,0.));
#8308=DIRECTION('',(0.,0.,-1.));
#8309=DIRECTION('center_axis',(0.,0.,-1.));
#8310=DIRECTION('ref_axis',(1.,0.,0.));
#8311=DIRECTION('center_axis',(0.,0.,-1.));
#8312=DIRECTION('ref_axis',(1.,0.,0.));
#8313=DIRECTION('center_axis',(0.,0.,1.));
#8314=DIRECTION('ref_axis',(1.,0.,0.));
#8315=DIRECTION('center_axis',(0.,0.,-1.));
#8316=DIRECTION('ref_axis',(1.,0.,0.));
#8317=DIRECTION('',(0.,0.,-1.));
#8318=DIRECTION('center_axis',(0.,0.,1.));
#8319=DIRECTION('ref_axis',(1.,0.,0.));
#8320=DIRECTION('center_axis',(0.,0.,-1.));
#8321=DIRECTION('ref_axis',(1.,0.,0.));
#8322=DIRECTION('',(0.,0.,-1.));
#8323=DIRECTION('center_axis',(0.,0.,1.));
#8324=DIRECTION('ref_axis',(1.,0.,0.));
#8325=DIRECTION('center_axis',(0.,-1.,0.));
#8326=DIRECTION('ref_axis',(-1.,0.,0.));
#8327=DIRECTION('',(0.0523359562429438,0.,0.998629534754574));
#8328=DIRECTION('',(1.,0.,0.));
#8329=DIRECTION('',(-0.0523359562429438,0.,-0.998629534754574));
#8330=DIRECTION('',(1.,0.,0.));
#8331=DIRECTION('center_axis',(0.,-1.,0.));
#8332=DIRECTION('ref_axis',(-1.,0.,0.));
#8333=DIRECTION('',(0.,0.,-1.));
#8334=DIRECTION('',(1.,0.,0.));
#8335=DIRECTION('',(0.,0.,1.));
#8336=DIRECTION('',(1.,0.,0.));
#8337=DIRECTION('center_axis',(0.,-1.,0.));
#8338=DIRECTION('ref_axis',(-1.,0.,0.));
#8339=DIRECTION('',(0.,0.,-1.));
#8340=DIRECTION('',(1.,0.,0.));
#8341=DIRECTION('',(0.,0.,1.));
#8342=DIRECTION('',(1.,0.,0.));
#8343=DIRECTION('center_axis',(0.,-1.,0.));
#8344=DIRECTION('ref_axis',(-1.,0.,0.));
#8345=DIRECTION('',(0.,0.,-1.));
#8346=DIRECTION('',(1.,0.,0.));
#8347=DIRECTION('',(0.,0.,1.));
#8348=DIRECTION('',(1.,0.,0.));
#8349=DIRECTION('center_axis',(0.,1.,0.));
#8350=DIRECTION('ref_axis',(1.,0.,0.));
#8351=DIRECTION('',(-0.0523359562429438,0.,-0.998629534754574));
#8352=DIRECTION('',(-1.,0.,0.));
#8353=DIRECTION('',(0.0523359562429438,0.,0.998629534754574));
#8354=DIRECTION('',(-1.,0.,0.));
#8355=DIRECTION('center_axis',(0.,1.,0.));
#8356=DIRECTION('ref_axis',(1.,0.,0.));
#8357=DIRECTION('',(0.,0.,1.));
#8358=DIRECTION('',(-1.,0.,0.));
#8359=DIRECTION('',(0.,0.,-1.));
#8360=DIRECTION('',(-1.,0.,0.));
#8361=DIRECTION('center_axis',(0.,1.,0.));
#8362=DIRECTION('ref_axis',(1.,0.,0.));
#8363=DIRECTION('',(0.,0.,1.));
#8364=DIRECTION('',(-1.,0.,0.));
#8365=DIRECTION('',(0.,0.,-1.));
#8366=DIRECTION('',(-1.,0.,0.));
#8367=DIRECTION('center_axis',(0.,0.,1.));
#8368=DIRECTION('ref_axis',(1.,0.,0.));
#8369=DIRECTION('center_axis',(0.,0.,1.));
#8370=DIRECTION('ref_axis',(1.,0.,0.));
#8371=DIRECTION('center_axis',(0.,0.,1.));
#8372=DIRECTION('ref_axis',(1.,0.,0.));
#8373=DIRECTION('center_axis',(0.,0.,1.));
#8374=DIRECTION('ref_axis',(1.,0.,0.));
#8375=DIRECTION('center_axis',(0.,0.,1.));
#8376=DIRECTION('ref_axis',(1.,0.,0.));
#8377=DIRECTION('',(0.,1.,0.));
#8378=DIRECTION('',(0.,-1.,0.));
#8379=DIRECTION('center_axis',(0.,0.,1.));
#8380=DIRECTION('ref_axis',(1.,0.,0.));
#8381=DIRECTION('',(0.,-1.,0.));
#8382=DIRECTION('',(0.,1.,0.));
#8383=DIRECTION('center_axis',(0.,0.,1.));
#8384=DIRECTION('ref_axis',(1.,0.,0.));
#8385=DIRECTION('',(0.,-1.,0.));
#8386=DIRECTION('',(0.,1.,0.));
#8387=DIRECTION('center_axis',(0.,0.,1.));
#8388=DIRECTION('ref_axis',(1.,0.,0.));
#8389=DIRECTION('',(0.,-1.,0.));
#8390=DIRECTION('',(-1.,0.,0.));
#8391=DIRECTION('',(0.,1.,0.));
#8392=DIRECTION('center_axis',(0.,1.,0.));
#8393=DIRECTION('ref_axis',(1.,0.,0.));
#8394=DIRECTION('',(0.,0.,1.));
#8395=DIRECTION('',(-1.,0.,0.));
#8396=DIRECTION('',(0.,0.,-1.));
#8397=DIRECTION('center_axis',(-1.,0.,0.));
#8398=DIRECTION('ref_axis',(0.,-1.,0.));
#8399=DIRECTION('',(0.,-1.,0.));
#8400=DIRECTION('',(0.,-1.,1.26069923670246E-19));
#8401=DIRECTION('center_axis',(1.,0.,0.));
#8402=DIRECTION('ref_axis',(0.,1.,0.));
#8403=DIRECTION('',(0.,1.,0.));
#8404=DIRECTION('',(0.,1.,-1.26069923670246E-19));
#8405=DIRECTION('',(0.,1.,0.));
#8406=DIRECTION('center_axis',(1.,0.,0.));
#8407=DIRECTION('ref_axis',(0.,1.,0.));
#8408=DIRECTION('',(0.,1.,0.));
#8409=DIRECTION('',(0.,1.,-1.26069923670246E-19));
#8410=DIRECTION('',(0.,1.,0.));
#8411=DIRECTION('center_axis',(1.,0.,0.));
#8412=DIRECTION('ref_axis',(0.,1.,0.));
#8413=DIRECTION('',(0.,1.,0.));
#8414=DIRECTION('',(0.,1.,-1.26069923670246E-19));
#8415=DIRECTION('',(0.,1.,0.));
#8416=DIRECTION('center_axis',(0.998629534754574,0.,-0.0523359562429438));
#8417=DIRECTION('ref_axis',(-0.0523359562429438,0.,-0.998629534754574));
#8418=DIRECTION('',(0.,-1.,0.));
#8419=DIRECTION('',(6.6070447339401E-21,-1.,1.26069923670246E-19));
#8420=DIRECTION('',(0.,-1.,0.));
#8421=DIRECTION('center_axis',(0.,0.,1.));
#8422=DIRECTION('ref_axis',(1.,0.,0.));
#8423=DIRECTION('',(0.,-1.,0.));
#8424=DIRECTION('',(0.,-1.,0.));
#8425=DIRECTION('',(0.,-1.,0.));
#8426=DIRECTION('',(0.,1.,0.));
#8427=DIRECTION('',(0.,-1.,0.));
#8428=DIRECTION('',(0.,1.,0.));
#8429=DIRECTION('',(0.,-1.,0.));
#8430=DIRECTION('',(0.,-1.,0.));
#8431=DIRECTION('',(0.,-1.,0.));
#8432=DIRECTION('',(0.,1.,0.));
#8433=DIRECTION('',(0.,1.,0.));
#8434=DIRECTION('center_axis',(0.,0.,1.));
#8435=DIRECTION('ref_axis',(1.,0.,0.));
#8436=DIRECTION('center_axis',(-1.01338750660366E-31,1.26069923670246E-19,
1.));
#8437=DIRECTION('ref_axis',(1.,0.,0.));
#8438=DIRECTION('',(0.,0.,-1.));
#8439=DIRECTION('center_axis',(0.,0.,1.));
#8440=DIRECTION('ref_axis',(1.,0.,0.));
#8441=DIRECTION('center_axis',(-1.01338750660366E-31,1.26069923670246E-19,
1.));
#8442=DIRECTION('ref_axis',(1.,0.,0.));
#8443=DIRECTION('',(0.,0.,-1.));
#8444=DIRECTION('center_axis',(1.,0.,0.));
#8445=DIRECTION('ref_axis',(0.,1.,0.));
#8446=DIRECTION('',(0.,1.,-1.26069923670246E-19));
#8447=DIRECTION('center_axis',(0.995216631131787,0.0976926666577189,1.18580395612125E-14));
#8448=DIRECTION('ref_axis',(0.0975341006448478,-0.993601284365854,0.0569524970297685));
#8449=DIRECTION('center_axis',(-1.01338750660366E-31,1.26069923670246E-19,
1.));
#8450=DIRECTION('ref_axis',(1.,0.,1.01338750660366E-31));
#8451=DIRECTION('center_axis',(-1.01338750660366E-31,1.26069923670246E-19,
1.));
#8452=DIRECTION('ref_axis',(1.,0.,1.01338750660366E-31));
#8453=DIRECTION('',(-6.60704473394009E-21,-1.,1.26069923670246E-19));
#8454=DIRECTION('center_axis',(-1.,0.,0.));
#8455=DIRECTION('ref_axis',(0.,-1.,0.));
#8456=DIRECTION('',(0.,-1.,1.26069923670246E-19));
#8457=DIRECTION('center_axis',(-1.01338750660366E-31,1.26069923670246E-19,
1.));
#8458=DIRECTION('ref_axis',(1.,0.,1.01338750660366E-31));
#8459=DIRECTION('center_axis',(-1.,0.,0.));
#8460=DIRECTION('ref_axis',(0.,-1.,0.));
#8461=DIRECTION('',(0.,-1.,1.26069923670246E-19));
#8462=DIRECTION('center_axis',(-1.01338750660366E-31,1.26069923670246E-19,
1.));
#8463=DIRECTION('ref_axis',(1.,0.,1.01338750660366E-31));
#8464=DIRECTION('center_axis',(-1.,0.,0.));
#8465=DIRECTION('ref_axis',(0.,-1.,0.));
#8466=DIRECTION('',(0.,-1.,1.26069923670246E-19));
#8467=DIRECTION('center_axis',(-0.982258063247475,0.187534256031586,1.45403402392141E-15));
#8468=DIRECTION('ref_axis',(1.48029736616688E-15,0.,1.));
#8469=DIRECTION('center_axis',(-1.01338750660366E-31,1.26069923670246E-19,
1.));
#8470=DIRECTION('ref_axis',(1.,0.,1.01338750660366E-31));
#8471=DIRECTION('',(-6.6070447339401E-21,1.,-1.26069923670246E-19));
#8472=DIRECTION('center_axis',(-0.982258063247479,-0.187534256031562,9.14061384143289E-15));
#8473=DIRECTION('ref_axis',(-0.187187393251729,0.980441281772238,0.0607928680392112));
#8474=DIRECTION('center_axis',(-0.45173408531537,0.373496730537872,-0.810207694632559));
#8475=DIRECTION('ref_axis',(-0.624418441188311,0.516273298501642,0.586142893463867));
#8476=DIRECTION('center_axis',(-2.96465769266614E-15,1.,0.));
#8477=DIRECTION('ref_axis',(0.,0.,1.));
#8478=DIRECTION('center_axis',(0.0522655346583812,-0.0518587053130894,0.997285810873755));
#8479=DIRECTION('ref_axis',(-0.998629534754574,0.,0.0523359562429445));
#8480=DIRECTION('center_axis',(0.377681861983732,-0.843372107574977,0.38220400219391));
#8481=DIRECTION('ref_axis',(0.592794689304902,0.537329962094562,0.599892463836113));
#8482=DIRECTION('center_axis',(0.995216631131786,-0.0976926666577302,0.));
#8483=DIRECTION('ref_axis',(0.,0.,1.));
#8484=DIRECTION('center_axis',(-0.0522650609395843,-0.052032719242908,0.997276771780618));
#8485=DIRECTION('ref_axis',(0.0975341006448596,0.993601284365853,0.0569524970297681));
#8486=DIRECTION('center_axis',(1.55158195278682E-16,1.,-2.96059473233375E-15));
#8487=DIRECTION('ref_axis',(0.998629534754574,0.,0.0523359562429438));
#8488=DIRECTION('center_axis',(-0.45173408531537,-0.373496730537869,-0.810207694632561));
#8489=DIRECTION('ref_axis',(-0.624418441188315,-0.516273298501641,0.586142893463864));
#8490=DIRECTION('center_axis',(0.0522655346583823,0.0518587053130918,0.997285810873755));
#8491=DIRECTION('ref_axis',(-0.187187393251729,-0.980441281772238,0.0607928680392122));
#8492=DIRECTION('center_axis',(-2.71526841737693E-16,-1.,-5.18104078158406E-15));
#8493=DIRECTION('ref_axis',(-0.998629534754574,0.,0.0523359562429439));
#8494=DIRECTION('center_axis',(-6.6070447339401E-21,1.,-1.26069923670246E-19));
#8495=DIRECTION('ref_axis',(-0.688354575693753,0.,0.725374371012289));
#8496=DIRECTION('center_axis',(-0.377681861983722,-0.843372107574983,-0.382204002193908));
#8497=DIRECTION('ref_axis',(0.592794689304909,-0.537329962094554,0.599892463836112));
#8498=DIRECTION('center_axis',(-0.0522650609395818,0.0520327192429072,0.997276771780618));
#8499=DIRECTION('ref_axis',(0.998629534754574,0.,0.0523359562429431));
#8500=DIRECTION('center_axis',(2.96465769266612E-15,-1.,0.));
#8501=DIRECTION('ref_axis',(0.,0.,1.));
#8502=DIRECTION('center_axis',(-6.60704473394009E-21,-1.,1.26069923670246E-19));
#8503=DIRECTION('ref_axis',(0.688354575693758,0.,0.725374371012284));
#8504=DIRECTION('',(6.60704473394009E-21,1.,-1.26069923670246E-19));
#8505=DIRECTION('center_axis',(-0.998629534754574,0.,-0.0523359562429438));
#8506=DIRECTION('ref_axis',(-0.0523359562429438,0.,0.998629534754574));
#8507=DIRECTION('center_axis',(-0.45173408531537,0.373496730537872,-0.81020769463256));
#8508=DIRECTION('ref_axis',(-0.624418441188311,0.516273298501643,0.586142893463866));
#8509=DIRECTION('center_axis',(-2.96465769266614E-15,1.,0.));
#8510=DIRECTION('ref_axis',(0.,0.,1.));
#8511=DIRECTION('center_axis',(-0.982258063247479,-0.187534256031562,9.14061384143289E-15));
#8512=DIRECTION('ref_axis',(-0.187187393251729,0.980441281772238,0.0607928680392111));
#8513=DIRECTION('center_axis',(0.0522655346583812,-0.0518587053130894,0.997285810873755));
#8514=DIRECTION('ref_axis',(-0.998629534754574,0.,0.0523359562429445));
#8515=DIRECTION('center_axis',(0.377681861983731,-0.843372107574978,0.38220400219391));
#8516=DIRECTION('ref_axis',(0.592794689304906,0.537329962094559,0.599892463836111));
#8517=DIRECTION('center_axis',(0.995216631131786,-0.0976926666577302,0.));
#8518=DIRECTION('ref_axis',(0.,0.,1.));
#8519=DIRECTION('center_axis',(1.55158195278682E-16,1.,-2.96059473233375E-15));
#8520=DIRECTION('ref_axis',(0.998629534754574,0.,0.0523359562429438));
#8521=DIRECTION('center_axis',(-0.0522650609395843,-0.052032719242908,0.997276771780618));
#8522=DIRECTION('ref_axis',(0.0975341006448596,0.993601284365853,0.0569524970297681));
#8523=DIRECTION('center_axis',(-0.45173408531537,-0.373496730537868,-0.810207694632561));
#8524=DIRECTION('ref_axis',(-0.624418441188315,-0.516273298501641,0.586142893463864));
#8525=DIRECTION('center_axis',(-0.982258063247475,0.187534256031586,1.45403402392141E-15));
#8526=DIRECTION('ref_axis',(1.48029736616688E-15,0.,1.));
#8527=DIRECTION('center_axis',(-2.71526841737693E-16,-1.,-5.18104078158406E-15));
#8528=DIRECTION('ref_axis',(-0.998629534754574,0.,0.0523359562429439));
#8529=DIRECTION('center_axis',(0.0522655346583823,0.0518587053130918,0.997285810873755));
#8530=DIRECTION('ref_axis',(-0.187187393251729,-0.980441281772238,0.0607928680392122));
#8531=DIRECTION('center_axis',(-6.6070447339401E-21,1.,-1.26069923670246E-19));
#8532=DIRECTION('ref_axis',(-0.688354575693753,0.,0.725374371012289));
#8533=DIRECTION('',(6.6070447339401E-21,-1.,1.26069923670246E-19));
#8534=DIRECTION('',(-6.6070447339401E-21,1.,-1.26069923670246E-19));
#8535=DIRECTION('center_axis',(-0.377681861983727,-0.843372107574981,-0.382204002193907));
#8536=DIRECTION('ref_axis',(0.592794689304909,-0.537329962094554,0.599892463836112));
#8537=DIRECTION('center_axis',(-0.0522650609395818,0.0520327192429072,0.997276771780618));
#8538=DIRECTION('ref_axis',(0.998629534754574,0.,0.0523359562429431));
#8539=DIRECTION('center_axis',(2.96465769266612E-15,-1.,0.));
#8540=DIRECTION('ref_axis',(0.,0.,1.));
#8541=DIRECTION('center_axis',(0.995216631131787,0.0976926666577189,1.18580395612125E-14));
#8542=DIRECTION('ref_axis',(0.0975341006448478,-0.993601284365854,0.0569524970297685));
#8543=DIRECTION('center_axis',(-6.60704473394009E-21,-1.,1.26069923670246E-19));
#8544=DIRECTION('ref_axis',(0.688354575693758,0.,0.725374371012284));
#8545=DIRECTION('',(6.60704473394009E-21,1.,-1.26069923670246E-19));
#8546=DIRECTION('',(-6.60704473394009E-21,-1.,1.26069923670246E-19));
#8547=DIRECTION('center_axis',(0.998629534754574,0.,-0.0523359562429438));
#8548=DIRECTION('ref_axis',(-0.0523359562429438,0.,-0.998629534754574));
#8549=DIRECTION('center_axis',(-1.01338750660366E-31,1.26069923670246E-19,
1.));
#8550=DIRECTION('ref_axis',(1.,0.,1.01338750660366E-31));
#8551=DIRECTION('center_axis',(-0.998629534754574,0.,-0.0523359562429438));
#8552=DIRECTION('ref_axis',(-0.0523359562429438,0.,0.998629534754574));
#9812=CARTESIAN_POINT('',(0.,0.,0.));
#9813=CARTESIAN_POINT('Origin',(9.,-1.,0.8));
#9814=CARTESIAN_POINT('',(8.85,-1.,0.9));
#9815=CARTESIAN_POINT('Origin',(9.,-1.,0.9));
#9816=CARTESIAN_POINT('',(8.85,-1.,0.7));
#9817=CARTESIAN_POINT('',(8.85,-1.,0.8));
#9818=CARTESIAN_POINT('Origin',(9.,-1.,0.7));
#9819=CARTESIAN_POINT('Origin',(3.,-1.,0.8));
#9820=CARTESIAN_POINT('',(2.85,-1.,0.9));
#9821=CARTESIAN_POINT('Origin',(3.,-1.,0.9));
#9822=CARTESIAN_POINT('',(2.85,-1.,0.7));
#9823=CARTESIAN_POINT('',(2.85,-1.,0.8));
#9824=CARTESIAN_POINT('Origin',(3.,-1.,0.7));
#9825=CARTESIAN_POINT('Origin',(3.,1.,0.8));
#9826=CARTESIAN_POINT('',(2.85,1.,0.9));
#9827=CARTESIAN_POINT('Origin',(3.,1.,0.9));
#9828=CARTESIAN_POINT('',(2.85,1.,0.7));
#9829=CARTESIAN_POINT('',(2.85,1.,0.8));
#9830=CARTESIAN_POINT('Origin',(3.,1.,0.7));
#9831=CARTESIAN_POINT('Origin',(9.,1.,0.8));
#9832=CARTESIAN_POINT('',(8.85,1.,0.9));
#9833=CARTESIAN_POINT('Origin',(9.,1.,0.9));
#9834=CARTESIAN_POINT('',(8.85,1.,0.7));
#9835=CARTESIAN_POINT('',(8.85,1.,0.8));
#9836=CARTESIAN_POINT('Origin',(9.,1.,0.7));
#9837=CARTESIAN_POINT('Origin',(2.,0.,0.75));
#9838=CARTESIAN_POINT('',(1.7,3.67394039744206E-17,0.9));
#9839=CARTESIAN_POINT('Origin',(2.,0.,0.9));
#9840=CARTESIAN_POINT('',(1.7,3.67394039744206E-17,0.6));
#9841=CARTESIAN_POINT('',(1.7,3.67394039744206E-17,0.75));
#9842=CARTESIAN_POINT('Origin',(2.,0.,0.6));
#9843=CARTESIAN_POINT('Origin',(2.,0.,0.6));
#9844=CARTESIAN_POINT('',(1.83,-2.0818995585505E-17,0.6));
#9845=CARTESIAN_POINT('Origin',(2.,0.,0.6));
#9846=CARTESIAN_POINT('Origin',(10.,0.,0.75));
#9847=CARTESIAN_POINT('',(9.7,3.67394039744206E-17,0.9));
#9848=CARTESIAN_POINT('Origin',(10.,0.,0.9));
#9849=CARTESIAN_POINT('',(9.7,3.67394039744206E-17,0.6));
#9850=CARTESIAN_POINT('',(9.7,3.67394039744206E-17,0.75));
#9851=CARTESIAN_POINT('Origin',(10.,0.,0.6));
#9852=CARTESIAN_POINT('Origin',(10.,0.,0.6));
#9853=CARTESIAN_POINT('',(9.83,-2.0818995585505E-17,0.6));
#9854=CARTESIAN_POINT('Origin',(10.,0.,0.6));
#9855=CARTESIAN_POINT('Origin',(2.,0.,0.45));
#9856=CARTESIAN_POINT('',(1.83,-2.0818995585505E-17,0.32));
#9857=CARTESIAN_POINT('',(1.83,2.0818995585505E-17,0.45));
#9858=CARTESIAN_POINT('Origin',(2.,0.,0.32));
#9859=CARTESIAN_POINT('Origin',(10.,0.,0.45));
#9860=CARTESIAN_POINT('',(9.83,-2.0818995585505E-17,0.32));
#9861=CARTESIAN_POINT('',(9.83,2.0818995585505E-17,0.45));
#9862=CARTESIAN_POINT('Origin',(10.,0.,0.32));
#9863=CARTESIAN_POINT('Origin',(11.2,-0.62,0.32));
#9864=CARTESIAN_POINT('',(0.200274469199584,-0.62,0.));
#9865=CARTESIAN_POINT('',(0.217044958570157,-0.62,0.32));
#9866=CARTESIAN_POINT('',(0.223426876981161,-0.62,0.441774257530303));
#9867=CARTESIAN_POINT('',(0.,-0.62,0.));
#9868=CARTESIAN_POINT('',(8.63987299740311,-0.62,0.));
#9869=CARTESIAN_POINT('',(0.0167704893705732,-0.62,0.32));
#9870=CARTESIAN_POINT('',(0.0237009700302462,-0.62,0.452241448778892));
#9871=CARTESIAN_POINT('',(-0.1,-0.62,0.32));
#9872=CARTESIAN_POINT('Origin',(11.2,-0.62,0.32));
#9873=CARTESIAN_POINT('',(0.9,-0.62,0.32));
#9874=CARTESIAN_POINT('',(0.9,-0.62,0.));
#9875=CARTESIAN_POINT('',(0.9,-0.62,0.16));
#9876=CARTESIAN_POINT('',(1.1,-0.62,0.32));
#9877=CARTESIAN_POINT('',(-0.1,-0.62,0.32));
#9878=CARTESIAN_POINT('',(1.1,-0.62,0.));
#9879=CARTESIAN_POINT('',(1.1,-0.62,0.16));
#9880=CARTESIAN_POINT('',(8.63987299740311,-0.62,0.));
#9881=CARTESIAN_POINT('Origin',(11.2,-0.62,0.32));
#9882=CARTESIAN_POINT('',(3.9,-0.62,0.32));
#9883=CARTESIAN_POINT('',(3.9,-0.62,0.));
#9884=CARTESIAN_POINT('',(3.9,-0.62,0.16));
#9885=CARTESIAN_POINT('',(4.1,-0.62,0.32));
#9886=CARTESIAN_POINT('',(-0.1,-0.62,0.32));
#9887=CARTESIAN_POINT('',(4.1,-0.62,0.));
#9888=CARTESIAN_POINT('',(4.1,-0.62,0.16));
#9889=CARTESIAN_POINT('',(8.63987299740311,-0.62,0.));
#9890=CARTESIAN_POINT('Origin',(11.2,-0.62,0.32));
#9891=CARTESIAN_POINT('',(7.9,-0.62,0.32));
#9892=CARTESIAN_POINT('',(7.9,-0.62,0.));
#9893=CARTESIAN_POINT('',(7.9,-0.62,0.16));
#9894=CARTESIAN_POINT('',(8.1,-0.62,0.32));
#9895=CARTESIAN_POINT('',(-0.1,-0.62,0.32));
#9896=CARTESIAN_POINT('',(8.1,-0.62,0.));
#9897=CARTESIAN_POINT('',(8.1,-0.62,0.16));
#9898=CARTESIAN_POINT('',(8.63987299740311,-0.62,0.));
#9899=CARTESIAN_POINT('Origin',(-0.0999999999999996,0.62,0.32));
#9900=CARTESIAN_POINT('',(0.217044958570158,0.62,0.32));
#9901=CARTESIAN_POINT('',(0.200274469199586,0.62,0.));
#9902=CARTESIAN_POINT('',(0.207951231396534,0.62,0.146481348799182));
#9903=CARTESIAN_POINT('',(0.0167704893705736,0.62,0.32));
#9904=CARTESIAN_POINT('',(11.2,0.62,0.32));
#9905=CARTESIAN_POINT('',(0.,0.62,0.));
#9906=CARTESIAN_POINT('',(0.00822532444561912,0.62,0.156948540047771));
#9907=CARTESIAN_POINT('',(2.98987299740311,0.62,0.));
#9908=CARTESIAN_POINT('Origin',(-0.0999999999999996,0.62,0.32));
#9909=CARTESIAN_POINT('',(0.9,0.62,0.));
#9910=CARTESIAN_POINT('',(0.9,0.62,0.32));
#9911=CARTESIAN_POINT('',(0.9,0.62,0.16));
#9912=CARTESIAN_POINT('',(1.1,0.62,0.));
#9913=CARTESIAN_POINT('',(2.98987299740311,0.62,0.));
#9914=CARTESIAN_POINT('',(1.1,0.62,0.32));
#9915=CARTESIAN_POINT('',(1.1,0.62,0.16));
#9916=CARTESIAN_POINT('',(11.2,0.62,0.32));
#9917=CARTESIAN_POINT('Origin',(-0.0999999999999996,0.62,0.32));
#9918=CARTESIAN_POINT('',(3.9,0.62,0.));
#9919=CARTESIAN_POINT('',(3.9,0.62,0.32));
#9920=CARTESIAN_POINT('',(3.9,0.62,0.16));
#9921=CARTESIAN_POINT('',(4.1,0.62,0.));
#9922=CARTESIAN_POINT('',(2.98987299740311,0.62,0.));
#9923=CARTESIAN_POINT('',(4.1,0.62,0.32));
#9924=CARTESIAN_POINT('',(4.1,0.62,0.16));
#9925=CARTESIAN_POINT('',(11.2,0.62,0.32));
#9926=CARTESIAN_POINT('Origin',(5.55,0.,0.32));
#9927=CARTESIAN_POINT('',(1.6,-4.89858719658941E-17,0.32));
#9928=CARTESIAN_POINT('Origin',(2.,0.,0.32));
#9929=CARTESIAN_POINT('Origin',(5.55,0.,0.32));
#9930=CARTESIAN_POINT('',(9.6,-4.89858719658942E-17,0.32));
#9931=CARTESIAN_POINT('Origin',(10.,0.,0.32));
#9932=CARTESIAN_POINT('Origin',(5.55,0.,0.32));
#9933=CARTESIAN_POINT('',(0.217044958570157,-0.7,0.32));
#9934=CARTESIAN_POINT('',(0.0167704893705731,-0.7,0.32));
#9935=CARTESIAN_POINT('Origin',(5.55,0.,0.32));
#9936=CARTESIAN_POINT('',(0.9,0.724814814814815,0.32));
#9937=CARTESIAN_POINT('',(1.1,-0.724814814814815,0.32));
#9938=CARTESIAN_POINT('Origin',(5.55,0.,0.32));
#9939=CARTESIAN_POINT('',(3.9,0.883148148148148,0.32));
#9940=CARTESIAN_POINT('',(4.1,-0.883148148148148,0.32));
#9941=CARTESIAN_POINT('Origin',(5.55,0.,0.32));
#9942=CARTESIAN_POINT('',(7.9,0.62,0.32));
#9943=CARTESIAN_POINT('',(7.9,0.886851851851852,0.32));
#9944=CARTESIAN_POINT('',(8.1,0.62,0.32));
#9945=CARTESIAN_POINT('',(11.2,0.62,0.32));
#9946=CARTESIAN_POINT('',(8.1,-0.886851851851852,0.32));
#9947=CARTESIAN_POINT('Origin',(-0.0999999999999996,0.62,0.32));
#9948=CARTESIAN_POINT('',(7.9,0.62,0.));
#9949=CARTESIAN_POINT('',(7.9,0.62,0.16));
#9950=CARTESIAN_POINT('',(8.1,0.62,0.));
#9951=CARTESIAN_POINT('',(2.98987299740311,0.62,0.));
#9952=CARTESIAN_POINT('',(8.1,0.62,0.16));
#9953=CARTESIAN_POINT('Origin',(11.2,1.53779953703704,0.));
#9954=CARTESIAN_POINT('',(11.2,1.47592264243751,0.));
#9955=CARTESIAN_POINT('',(11.2,-1.47592264243751,0.));
#9956=CARTESIAN_POINT('',(11.2,1.53779953703704,0.));
#9957=CARTESIAN_POINT('',(11.2,-1.44160695250311,0.605635447211793));
#9958=CARTESIAN_POINT('Ctrl Pts',(11.2,-1.44160695250311,0.605635447211793));
#9959=CARTESIAN_POINT('Ctrl Pts',(11.2,-1.44733381480461,0.504614841520655));
#9960=CARTESIAN_POINT('Ctrl Pts',(11.2,-1.45305922122436,0.403593539811385));
#9961=CARTESIAN_POINT('Ctrl Pts',(11.2,-1.46449774781658,0.201715464978033));
#9962=CARTESIAN_POINT('Ctrl Pts',(11.2,-1.47021094199039,0.100857470386242));
#9963=CARTESIAN_POINT('Ctrl Pts',(11.2,-1.47592264243751,0.));
#9964=CARTESIAN_POINT('',(11.2,-1.3413305091784,0.7));
#9965=CARTESIAN_POINT('Ctrl Pts',(11.2,-1.34133050917871,0.7));
#9966=CARTESIAN_POINT('Ctrl Pts',(11.2,-1.34927184579059,0.7));
#9967=CARTESIAN_POINT('Ctrl Pts',(11.1999981201149,-1.35715077597425,0.699006225306896));
#9968=CARTESIAN_POINT('Ctrl Pts',(11.1999964866412,-1.36482619101963,0.697118463987577));
#9969=CARTESIAN_POINT('Ctrl Pts',(11.1999955714568,-1.36912648693643,0.696060810134936));
#9970=CARTESIAN_POINT('Ctrl Pts',(11.1999947385598,-1.37336294684024,0.694721504600825));
#9971=CARTESIAN_POINT('Ctrl Pts',(11.1999942054834,-1.37750904339755,0.693111246644731));
#9972=CARTESIAN_POINT('Ctrl Pts',(11.1999932489192,-1.38494889279378,0.690221763364053));
#9973=CARTESIAN_POINT('Ctrl Pts',(11.1999934335488,-1.39201911070639,0.686493604183975));
#9974=CARTESIAN_POINT('Ctrl Pts',(11.1999946360439,-1.39857284316731,0.682006025455124));
#9975=CARTESIAN_POINT('Ctrl Pts',(11.1999952980149,-1.40218065925828,0.679535622697003));
#9976=CARTESIAN_POINT('Ctrl Pts',(11.1999962427007,-1.40563167682227,0.676834205328214));
#9977=CARTESIAN_POINT('Ctrl Pts',(11.1999970766466,-1.40889738828709,0.673909521834337));
#9978=CARTESIAN_POINT('Ctrl Pts',(11.1999978839828,-1.41205889660265,0.671078159882768));
#9979=CARTESIAN_POINT('Ctrl Pts',(11.1999985961359,-1.41502771690814,0.668054510912379));
#9980=CARTESIAN_POINT('Ctrl Pts',(11.1999985943254,-1.41778154893794,0.664849526385156));
#9981=CARTESIAN_POINT('Ctrl Pts',(11.1999985909468,-1.42292039881534,0.658868793295219));
#9982=CARTESIAN_POINT('Ctrl Pts',(11.1999963776609,-1.42731355725865,0.652257958652517));
#9983=CARTESIAN_POINT('Ctrl Pts',(11.1999956369,-1.43089859237711,0.645180832176479));
#9984=CARTESIAN_POINT('Ctrl Pts',(11.1999955610412,-1.43126572346771,0.644456088045497));
#9985=CARTESIAN_POINT('Ctrl Pts',(11.1999954968237,-1.43162433912915,0.643726434786758));
#9986=CARTESIAN_POINT('Ctrl Pts',(11.1999954455063,-1.43197434355081,0.642992037678167));
#9987=CARTESIAN_POINT('Ctrl Pts',(11.1999949451572,-1.43538691836834,0.635831599341589));
#9988=CARTESIAN_POINT('Ctrl Pts',(11.1999960935741,-1.43794480573841,0.628305806294037));
#9989=CARTESIAN_POINT('Ctrl Pts',(11.1999977538348,-1.43959303921538,0.620581877990282));
#9990=CARTESIAN_POINT('Ctrl Pts',(11.1999988103007,-1.44064185190664,0.615666946856702));
#9991=CARTESIAN_POINT('Ctrl Pts',(11.1999999935832,-1.44132148083109,0.610671141596651));
#9992=CARTESIAN_POINT('Ctrl Pts',(11.1999999950647,-1.44160695392865,0.605635447210179));
#9993=CARTESIAN_POINT('',(11.2,1.34133050917871,0.7));
#9994=CARTESIAN_POINT('',(11.2,0.768899768518519,0.7));
#9995=CARTESIAN_POINT('',(11.2,1.44160695250311,0.605635447211793));
#9996=CARTESIAN_POINT('Ctrl Pts',(11.1999999950647,1.44160695392865,0.605635447210179));
#9997=CARTESIAN_POINT('Ctrl Pts',(11.1999999927383,1.44115867123275,0.613543073794128));
#9998=CARTESIAN_POINT('Ctrl Pts',(11.199997327584,1.43974095598264,0.62135504174347));
#9999=CARTESIAN_POINT('Ctrl Pts',(11.1999961426836,1.43743894790867,0.628911795513178));
#10000=CARTESIAN_POINT('Ctrl Pts',(11.1999954950047,1.43618064644969,0.633042395401645));
#10001=CARTESIAN_POINT('Ctrl Pts',(11.1999951984378,1.4346571631488,0.63709676955888));
#10002=CARTESIAN_POINT('Ctrl Pts',(11.1999953420225,1.43287614971348,0.641047046155727));
#10003=CARTESIAN_POINT('Ctrl Pts',(11.1999956050472,1.42961361303411,0.648283331988978));
#10004=CARTESIAN_POINT('Ctrl Pts',(11.1999975633633,1.42552584716917,0.655091209244077));
#10005=CARTESIAN_POINT('Ctrl Pts',(11.1999983488166,1.42067941835906,0.661308913390503));
#10006=CARTESIAN_POINT('Ctrl Pts',(11.1999985007599,1.41974189284539,0.662511707551344));
#10007=CARTESIAN_POINT('Ctrl Pts',(11.1999985958742,1.41877583892185,0.663692344451305));
#10008=CARTESIAN_POINT('Ctrl Pts',(11.1999985956185,1.41778154881703,0.664849526385225));
#10009=CARTESIAN_POINT('Ctrl Pts',(11.199998595152,1.41596832836708,0.666959801783445));
#10010=CARTESIAN_POINT('Ctrl Pts',(11.1999982799021,1.41406123008998,0.668992111776222));
#10011=CARTESIAN_POINT('Ctrl Pts',(11.1999978412043,1.41206657472189,0.670943322037058));
#10012=CARTESIAN_POINT('Ctrl Pts',(11.1999965906985,1.40638082038708,0.676505236328724));
#10013=CARTESIAN_POINT('Ctrl Pts',(11.1999945592311,1.40005057587654,0.681348449922958));
#10014=CARTESIAN_POINT('Ctrl Pts',(11.1999938793032,1.39324090595796,0.685420973467861));
#10015=CARTESIAN_POINT('Ctrl Pts',(11.1999934424014,1.38886521116801,0.68803785802621));
#10016=CARTESIAN_POINT('Ctrl Pts',(11.1999934711477,1.38429057260668,0.690335857752236));
#10017=CARTESIAN_POINT('Ctrl Pts',(11.1999939665515,1.37955471147715,0.692291686537622));
#10018=CARTESIAN_POINT('Ctrl Pts',(11.1999947349645,1.37220899016913,0.695325342464331));
#10019=CARTESIAN_POINT('Ctrl Pts',(11.1999966395725,1.36455954597093,0.697503651902993));
#10020=CARTESIAN_POINT('Ctrl Pts',(11.1999981885915,1.35675452105021,0.698758058199902));
#10021=CARTESIAN_POINT('Ctrl Pts',(11.1999991983045,1.35166689148409,0.699575730741489));
#10022=CARTESIAN_POINT('Ctrl Pts',(11.2,1.34651254223162,0.7));
#10023=CARTESIAN_POINT('Ctrl Pts',(11.2,1.34133050917871,0.7));
#10024=CARTESIAN_POINT('Ctrl Pts',(11.2,1.47592264243751,0.));
#10025=CARTESIAN_POINT('Ctrl Pts',(11.2,1.47021025951677,0.100869521536925));
#10026=CARTESIAN_POINT('Ctrl Pts',(11.2,1.4644963825062,0.20173956751342));
#10027=CARTESIAN_POINT('Ctrl Pts',(11.2,1.45305785520703,0.403617642353031));
#10028=CARTESIAN_POINT('Ctrl Pts',(11.2,1.44733313162379,0.50462689268162));
#10029=CARTESIAN_POINT('Ctrl Pts',(11.2,1.44160695250311,0.605635447211793));
#10030=CARTESIAN_POINT('Origin',(8.1,-1.7737037037037,0.));
#10031=CARTESIAN_POINT('',(8.1,1.69866351109718,0.));
#10032=CARTESIAN_POINT('',(8.1,-1.7737037037037,0.));
#10033=CARTESIAN_POINT('',(8.1,1.66641703131627,0.605314487869832));
#10034=CARTESIAN_POINT('Ctrl Pts',(8.1,1.66641703131627,0.605314487869832));
#10035=CARTESIAN_POINT('Ctrl Pts',(8.1,1.67178339996556,0.504592280948055));
#10036=CARTESIAN_POINT('Ctrl Pts',(8.1,1.67714947719849,0.403869246528492));
#10037=CARTESIAN_POINT('Ctrl Pts',(8.1,1.68789827452893,0.202098297941347));
#10038=CARTESIAN_POINT('Ctrl Pts',(8.1,1.69328107955938,0.101048748975501));
#10039=CARTESIAN_POINT('Ctrl Pts',(8.1,1.69866351109718,0.));
#10040=CARTESIAN_POINT('',(8.1,1.56644778183753,0.7));
#10041=CARTESIAN_POINT('Ctrl Pts',(8.0999999986552,1.56644778212326,0.7));
#10042=CARTESIAN_POINT('Ctrl Pts',(8.10000000155239,1.57436337254628,0.699999999341293));
#10043=CARTESIAN_POINT('Ctrl Pts',(8.09999905041684,1.58221543358893,0.699005989267703));
#10044=CARTESIAN_POINT('Ctrl Pts',(8.09999821745812,1.58986365929578,0.697118696434997));
#10045=CARTESIAN_POINT('Ctrl Pts',(8.099997748439,1.59417019217574,0.69605600700222));
#10046=CARTESIAN_POINT('Ctrl Pts',(8.09999731997616,1.59841215407948,0.694709061504878));
#10047=CARTESIAN_POINT('Ctrl Pts',(8.09999704681388,1.60256279759721,0.693088866918468));
#10048=CARTESIAN_POINT('Ctrl Pts',(8.09999655811104,1.60998853482381,0.690190246691698));
#10049=CARTESIAN_POINT('Ctrl Pts',(8.09999665589197,1.61704187682962,0.686451534538094));
#10050=CARTESIAN_POINT('Ctrl Pts',(8.09999726576867,1.62357667434142,0.681954089017224));
#10051=CARTESIAN_POINT('Ctrl Pts',(8.09999760196939,1.62717904774802,0.679474826559159));
#10052=CARTESIAN_POINT('Ctrl Pts',(8.09999808150314,1.6306235748906,0.676764109620253));
#10053=CARTESIAN_POINT('Ctrl Pts',(8.09999850764167,1.63388182210815,0.673830012183301));
#10054=CARTESIAN_POINT('Ctrl Pts',(8.09999892160867,1.637047006066,0.670979719520364));
#10055=CARTESIAN_POINT('Ctrl Pts',(8.09999928906958,1.640017230617,0.667935813742119));
#10056=CARTESIAN_POINT('Ctrl Pts',(8.09999928944056,1.64277007752663,0.664709670235875));
#10057=CARTESIAN_POINT('Ctrl Pts',(8.09999929012967,1.64788359851353,0.658716982277737));
#10058=CARTESIAN_POINT('Ctrl Pts',(8.09999816327153,1.65225000627493,0.652096887528603));
#10059=CARTESIAN_POINT('Ctrl Pts',(8.09999778355904,1.65580927004486,0.645014643130784));
#10060=CARTESIAN_POINT('Ctrl Pts',(8.09999774450894,1.65617530914943,0.644286296325024));
#10061=CARTESIAN_POINT('Ctrl Pts',(8.09999771143612,1.65653277094855,0.643553041785202));
#10062=CARTESIAN_POINT('Ctrl Pts',(8.0999976850083,1.65688156115921,0.642815048027137));
#10063=CARTESIAN_POINT('Ctrl Pts',(8.09999742811004,1.66027206465027,0.635641192980042));
#10064=CARTESIAN_POINT('Ctrl Pts',(8.09999800724182,1.66280786743682,0.628104262855387));
#10065=CARTESIAN_POINT('Ctrl Pts',(8.09999885110511,1.66443535430957,0.620372450280339));
#10066=CARTESIAN_POINT('Ctrl Pts',(8.09999939164969,1.6654778563549,0.615419764910946));
#10067=CARTESIAN_POINT('Ctrl Pts',(8.1,1.66614680274328,0.610386449940169));
#10068=CARTESIAN_POINT('Ctrl Pts',(8.1,1.66641703131627,0.605314487869832));
#10069=CARTESIAN_POINT('',(8.1,-1.56644778183827,0.7));
#10070=CARTESIAN_POINT('',(8.1,-0.886851851851852,0.7));
#10071=CARTESIAN_POINT('',(8.1,-1.66641703131627,0.605314487869832));
#10072=CARTESIAN_POINT('Ctrl Pts',(8.1,-1.66641703131627,0.605314487869832));
#10073=CARTESIAN_POINT('Ctrl Pts',(8.1,-1.66599546653325,0.613226902778437));
#10074=CARTESIAN_POINT('Ctrl Pts',(8.09999864563672,-1.66460605882141,0.621047760783158));
#10075=CARTESIAN_POINT('Ctrl Pts',(8.09999804140045,-1.66233302739118,0.628616817026045));
#10076=CARTESIAN_POINT('Ctrl Pts',(8.09999770486592,-1.66106704316887,0.632832467392296));
#10077=CARTESIAN_POINT('Ctrl Pts',(8.0999975536836,-1.65952595995304,0.636970042829054));
#10078=CARTESIAN_POINT('Ctrl Pts',(8.09999763427866,-1.65771765414013,0.640999885518982));
#10079=CARTESIAN_POINT('Ctrl Pts',(8.09999777898787,-1.65447082344915,0.64823550729937));
#10080=CARTESIAN_POINT('Ctrl Pts',(8.09999878245444,-1.65040085231772,0.655045563401426));
#10081=CARTESIAN_POINT('Ctrl Pts',(8.09999917121848,-1.64557198994432,0.661267087195486));
#10082=CARTESIAN_POINT('Ctrl Pts',(8.09999924425118,-1.6446648462537,0.662435854416292));
#10083=CARTESIAN_POINT('Ctrl Pts',(8.09999928944999,-1.64373079085321,0.663583781603691));
#10084=CARTESIAN_POINT('Ctrl Pts',(8.09999928890117,-1.64277007755202,0.664709670235858));
#10085=CARTESIAN_POINT('Ctrl Pts',(8.09999928782175,-1.64088054556816,0.666924069243459));
#10086=CARTESIAN_POINT('Ctrl Pts',(8.09999911129818,-1.63888792496677,0.66905326411728));
#10087=CARTESIAN_POINT('Ctrl Pts',(8.09999887085824,-1.63679941630975,0.671093569621172));
#10088=CARTESIAN_POINT('Ctrl Pts',(8.09999821641022,-1.6311147520694,0.676647030794692));
#10089=CARTESIAN_POINT('Ctrl Pts',(8.0999972000003,-1.62478663867955,0.681482189379454));
#10090=CARTESIAN_POINT('Ctrl Pts',(8.09999686812141,-1.6179789612855,0.685544965666037));
#10091=CARTESIAN_POINT('Ctrl Pts',(8.09999665686968,-1.61364565292072,0.68813105508359));
#10092=CARTESIAN_POINT('Ctrl Pts',(8.09999667786582,-1.6091170759025,0.690403516124292));
#10093=CARTESIAN_POINT('Ctrl Pts',(8.0999969341683,-1.60442977212996,0.692339085768374));
#10094=CARTESIAN_POINT('Ctrl Pts',(8.09999733452329,-1.59710801128849,0.695362524980696));
#10095=CARTESIAN_POINT('Ctrl Pts',(8.09999831212369,-1.58948382509795,0.697531565976904));
#10096=CARTESIAN_POINT('Ctrl Pts',(8.09999909563861,-1.58170429192971,0.698776637084609));
#10097=CARTESIAN_POINT('Ctrl Pts',(8.09999960249138,-1.57667174192468,0.69958206878261));
#10098=CARTESIAN_POINT('Ctrl Pts',(8.1000000005313,-1.5715735875011,0.699999999573449));
#10099=CARTESIAN_POINT('Ctrl Pts',(8.0999999986552,-1.56644778212326,0.7));
#10100=CARTESIAN_POINT('',(8.1,-1.69866351109718,0.));
#10101=CARTESIAN_POINT('Ctrl Pts',(8.1,-1.69866351109718,0.));
#10102=CARTESIAN_POINT('Ctrl Pts',(8.1,-1.69328105674055,0.101049177371948));
#10103=CARTESIAN_POINT('Ctrl Pts',(8.1,-1.68789822886868,0.202099155105557));
#10104=CARTESIAN_POINT('Ctrl Pts',(8.1,-1.67714943151225,0.403870104074094));
#10105=CARTESIAN_POINT('Ctrl Pts',(8.1,-1.67178337712185,0.50459270970527));
#10106=CARTESIAN_POINT('Ctrl Pts',(8.1,-1.66641703131627,0.605314487869832));
#10107=CARTESIAN_POINT('',(8.1,-1.7737037037037,0.));
#10108=CARTESIAN_POINT('Origin',(4.1,-1.7662962962963,0.));
#10109=CARTESIAN_POINT('',(4.1,1.70113889814581,0.));
#10110=CARTESIAN_POINT('',(4.1,-1.7662962962963,0.));
#10111=CARTESIAN_POINT('',(4.1,1.66887738702937,0.605315322680072));
#10112=CARTESIAN_POINT('Ctrl Pts',(4.1,1.66887738702937,0.605315322680072));
#10113=CARTESIAN_POINT('Ctrl Pts',(4.1,1.67424235111642,0.50466767694528));
#10114=CARTESIAN_POINT('Ctrl Pts',(4.1,1.67960699363804,0.404019058341251));
#10115=CARTESIAN_POINT('Ctrl Pts',(4.1,1.69036079691899,0.202247931921761));
#10116=CARTESIAN_POINT('Ctrl Pts',(4.1,1.6957500571643,0.101123491803998));
#10117=CARTESIAN_POINT('Ctrl Pts',(4.1,1.70113889814581,0.));
#10118=CARTESIAN_POINT('',(4.1,1.56887583540973,0.7));
#10119=CARTESIAN_POINT('Ctrl Pts',(4.1,1.56887583540973,0.7));
#10120=CARTESIAN_POINT('Ctrl Pts',(4.1,1.57679416129392,0.7));
#10121=CARTESIAN_POINT('Ctrl Pts',(4.10000107724674,1.58464912207822,0.699006028000541));
#10122=CARTESIAN_POINT('Ctrl Pts',(4.10000201939527,1.59230028572239,0.697118705459362));
#10123=CARTESIAN_POINT('Ctrl Pts',(4.10000255022779,1.59661116283941,0.696055335763773));
#10124=CARTESIAN_POINT('Ctrl Pts',(4.10000303435977,1.60085740028891,0.694707333985525));
#10125=CARTESIAN_POINT('Ctrl Pts',(4.10000334030352,1.60501217339351,0.693085708041268));
#10126=CARTESIAN_POINT('Ctrl Pts',(4.10000388718746,1.61243895913315,0.690187001388783));
#10127=CARTESIAN_POINT('Ctrl Pts',(4.10000376557609,1.61949349263125,0.686448444730844));
#10128=CARTESIAN_POINT('Ctrl Pts',(4.10000306534783,1.6260295229635,0.681951159450519));
#10129=CARTESIAN_POINT('Ctrl Pts',(4.10000267892397,1.62963645835533,0.679469313954069));
#10130=CARTESIAN_POINT('Ctrl Pts',(4.10000213012555,1.63308521926452,0.676755517937216));
#10131=CARTESIAN_POINT('Ctrl Pts',(4.1000016436875,1.63634725251217,0.673817835781739));
#10132=CARTESIAN_POINT('Ctrl Pts',(4.10000117237165,1.63950787692018,0.67097147916344));
#10133=CARTESIAN_POINT('Ctrl Pts',(4.10000075597222,1.64247408874941,0.667932078875657));
#10134=CARTESIAN_POINT('Ctrl Pts',(4.10000075698646,1.64522354659423,0.664710927554201));
#10135=CARTESIAN_POINT('Ctrl Pts',(4.1000007588733,1.65033845220459,0.658718515269377));
#10136=CARTESIAN_POINT('Ctrl Pts',(4.10000204656096,1.65470614797426,0.652098486008568));
#10137=CARTESIAN_POINT('Ctrl Pts',(4.10000248678323,1.65826650381873,0.645016049251367));
#10138=CARTESIAN_POINT('Ctrl Pts',(4.10000253228732,1.65863452415637,0.644283964909082));
#10139=CARTESIAN_POINT('Ctrl Pts',(4.10000257095464,1.65899387729575,0.643546919913709));
#10140=CARTESIAN_POINT('Ctrl Pts',(4.10000260201855,1.65934446736461,0.642805085364403));
#10141=CARTESIAN_POINT('Ctrl Pts',(4.10000290242009,1.66273482600052,0.635631222228741));
#10142=CARTESIAN_POINT('Ctrl Pts',(4.10000225562543,1.66527033938482,0.628094305374488));
#10143=CARTESIAN_POINT('Ctrl Pts',(4.10000130084992,1.66689736875237,0.62036252267401));
#10144=CARTESIAN_POINT('Ctrl Pts',(4.10000068968835,1.66793884687677,0.615413329558163));
#10145=CARTESIAN_POINT('Ctrl Pts',(4.09999999901039,1.66860722297681,0.610383627857512));
#10146=CARTESIAN_POINT('Ctrl Pts',(4.09999999630223,1.66887738567036,0.60531532268817));
#10147=CARTESIAN_POINT('',(4.1,-1.56887583540947,0.7));
#10148=CARTESIAN_POINT('',(4.1,-0.883148148148148,0.7));
#10149=CARTESIAN_POINT('',(4.1,-1.66887738702937,0.605315322680072));
#10150=CARTESIAN_POINT('Ctrl Pts',(4.09999999630223,-1.66887738567036,0.60531532268817));
#10151=CARTESIAN_POINT('Ctrl Pts',(4.10000000053001,-1.66845562780346,0.613227583070809));
#10152=CARTESIAN_POINT('Ctrl Pts',(4.10000153668442,-1.66706589531621,0.621048261667561));
#10153=CARTESIAN_POINT('Ctrl Pts',(4.10000221487211,-1.66479240287642,0.628617079688242));
#10154=CARTESIAN_POINT('Ctrl Pts',(4.10000259231836,-1.6635270876889,0.632829515245766));
#10155=CARTESIAN_POINT('Ctrl Pts',(4.10000275805793,-1.66198703315979,0.636963972243471));
#10156=CARTESIAN_POINT('Ctrl Pts',(4.10000266178038,-1.66018010017296,0.640990858692597));
#10157=CARTESIAN_POINT('Ctrl Pts',(4.10000248876893,-1.65693302887506,0.648227201990446));
#10158=CARTESIAN_POINT('Ctrl Pts',(4.10000134097948,-1.65286254930452,0.655037795911226));
#10159=CARTESIAN_POINT('Ctrl Pts',(4.100000893742,-1.6480330317196,0.661259713776781));
#10160=CARTESIAN_POINT('Ctrl Pts',(4.10000080951506,-1.647123502594,0.662431469633614));
#10161=CARTESIAN_POINT('Ctrl Pts',(4.10000075717637,-1.6461869221106,0.663582276554164));
#10162=CARTESIAN_POINT('Ctrl Pts',(4.10000075728519,-1.64522354661022,0.66471092755419));
#10163=CARTESIAN_POINT('Ctrl Pts',(4.10000075749815,-1.64333815989002,0.666919768869269));
#10164=CARTESIAN_POINT('Ctrl Pts',(4.1000009568795,-1.64135017761634,0.669043797975229));
#10165=CARTESIAN_POINT('Ctrl Pts',(4.10000122972053,-1.63926675509047,0.671079366787198));
#10166=CARTESIAN_POINT('Ctrl Pts',(4.10000197419082,-1.6335819569127,0.676633591976433));
#10167=CARTESIAN_POINT('Ctrl Pts',(4.10000313643093,-1.62725355063421,0.681469444454218));
#10168=CARTESIAN_POINT('Ctrl Pts',(4.1000035230587,-1.62044557755217,0.685533082105531));
#10169=CARTESIAN_POINT('Ctrl Pts',(4.10000376939409,-1.61610795658125,0.688122181633714));
#10170=CARTESIAN_POINT('Ctrl Pts',(4.10000375220654,-1.61157469281532,0.690397125746379));
#10171=CARTESIAN_POINT('Ctrl Pts',(4.10000346632868,-1.60688245467732,0.692334655286926));
#10172=CARTESIAN_POINT('Ctrl Pts',(4.10000302008581,-1.59955807566073,0.695359054367588));
#10173=CARTESIAN_POINT('Ctrl Pts',(4.1000019139068,-1.59193114173487,0.69752894708864));
#10174=CARTESIAN_POINT('Ctrl Pts',(4.10000102635309,-1.58414888227482,0.698774888159427));
#10175=CARTESIAN_POINT('Ctrl Pts',(4.10000045177616,-1.57911086966871,0.699581474839467));
#10176=CARTESIAN_POINT('Ctrl Pts',(4.1,-1.57400716417114,0.7));
#10177=CARTESIAN_POINT('Ctrl Pts',(4.1,-1.56887583540973,0.7));
#10178=CARTESIAN_POINT('',(4.1,-1.70113889814582,0.));
#10179=CARTESIAN_POINT('Ctrl Pts',(4.1,-1.70113889814582,0.));
#10180=CARTESIAN_POINT('Ctrl Pts',(4.1,-1.69575004793467,0.101123665001254));
#10181=CARTESIAN_POINT('Ctrl Pts',(4.1,-1.69036077845691,0.202248278345555));
#10182=CARTESIAN_POINT('Ctrl Pts',(4.1,-1.67960697517202,0.404019404791024));
#10183=CARTESIAN_POINT('Ctrl Pts',(4.1,-1.67424234188296,0.504667850166609));
#10184=CARTESIAN_POINT('Ctrl Pts',(4.1,-1.66887738702937,0.605315322680072));
#10185=CARTESIAN_POINT('',(4.1,-1.7662962962963,0.));
#10186=CARTESIAN_POINT('Origin',(1.1,-1.44962962962963,0.));
#10187=CARTESIAN_POINT('',(1.1,1.39262953588351,0.));
#10188=CARTESIAN_POINT('',(1.1,-1.44962962962963,0.));
#10189=CARTESIAN_POINT('',(1.10000000000005,1.35674377243284,0.605845626926786));
#10190=CARTESIAN_POINT('Ctrl Pts',(1.10000000000005,1.35674377243284,0.605845626926786));
#10191=CARTESIAN_POINT('Ctrl Pts',(1.10000000000005,1.36273568520883,0.504787121979256));
#10192=CARTESIAN_POINT('Ctrl Pts',(1.1,1.36872466312622,0.403727404115485));
#10193=CARTESIAN_POINT('Ctrl Pts',(1.1,1.38068651056748,0.201779555185378));
#10194=CARTESIAN_POINT('Ctrl Pts',(1.1,1.38665951284069,0.10088935150083));
#10195=CARTESIAN_POINT('Ctrl Pts',(1.1,1.39262953588351,0.));
#10196=CARTESIAN_POINT('',(1.1,1.25565664448622,0.7));
#10197=CARTESIAN_POINT('Ctrl Pts',(1.1,1.25565664448621,0.7));
#10198=CARTESIAN_POINT('Ctrl Pts',(1.1,1.26365753466764,0.700000000000001));
#10199=CARTESIAN_POINT('Ctrl Pts',(1.10000312127109,1.27160078819195,0.699008097631352));
#10200=CARTESIAN_POINT('Ctrl Pts',(1.10000579554281,1.27934333527045,0.697120485426804));
#10201=CARTESIAN_POINT('Ctrl Pts',(1.10000709386889,1.28310224676699,0.696204072889075));
#10202=CARTESIAN_POINT('Ctrl Pts',(1.10000828779753,1.28681383019745,0.695075712339665));
#10203=CARTESIAN_POINT('Ctrl Pts',(1.10000913303706,1.29046059826345,0.693742188764313));
#10204=CARTESIAN_POINT('Ctrl Pts',(1.10001087659788,1.29798315455626,0.69099139518989));
#10205=CARTESIAN_POINT('Ctrl Pts',(1.10001086910546,1.30515375246939,0.687398976275641));
#10206=CARTESIAN_POINT('Ctrl Pts',(1.10000899624477,1.31182501206943,0.683041610144935));
#10207=CARTESIAN_POINT('Ctrl Pts',(1.10000779407289,1.31610723164143,0.680244657298552));
#10208=CARTESIAN_POINT('Ctrl Pts',(1.10000585478529,1.32018349952736,0.677131483611404));
#10209=CARTESIAN_POINT('Ctrl Pts',(1.10000422180804,1.32400796947387,0.673713330684339));
#10210=CARTESIAN_POINT('Ctrl Pts',(1.10000291018178,1.3270798280974,0.670967830603965));
#10211=CARTESIAN_POINT('Ctrl Pts',(1.10000180047651,1.32997084712789,0.668041731908725));
#10212=CARTESIAN_POINT('Ctrl Pts',(1.10000182449184,1.33266034096938,0.664944387470286));
#10213=CARTESIAN_POINT('Ctrl Pts',(1.10000187074845,1.33784065079383,0.65897850512594));
#10214=CARTESIAN_POINT('Ctrl Pts',(1.10000564109429,1.34227630326151,0.652378581761819));
#10215=CARTESIAN_POINT('Ctrl Pts',(1.10000696187003,1.34590032739451,0.645305437365917));
#10216=CARTESIAN_POINT('Ctrl Pts',(1.100007110355,1.34630774940504,0.644510256482779));
#10217=CARTESIAN_POINT('Ctrl Pts',(1.10000723579819,1.34670486410349,0.643709073603569));
#10218=CARTESIAN_POINT('Ctrl Pts',(1.10000733566964,1.34709153749004,0.642902104572485));
#10219=CARTESIAN_POINT('Ctrl Pts',(1.10000822022419,1.35051627708745,0.63575483535061));
#10220=CARTESIAN_POINT('Ctrl Pts',(1.10000635568239,1.35308446649167,0.628241602461225));
#10221=CARTESIAN_POINT('Ctrl Pts',(1.10000361780323,1.35473867947858,0.620527690691125));
#10222=CARTESIAN_POINT('Ctrl Pts',(1.1000019043033,1.35577396762308,0.615699943921843));
#10223=CARTESIAN_POINT('Ctrl Pts',(1.09999998677418,1.35645041192828,0.610792997969602));
#10224=CARTESIAN_POINT('Ctrl Pts',(1.09999997754868,1.35674374570294,0.605845627052288));
#10225=CARTESIAN_POINT('',(1.1,-1.25565664448622,0.7));
#10226=CARTESIAN_POINT('',(1.1,-0.724814814814815,0.7));
#10227=CARTESIAN_POINT('',(1.10000000000005,-1.35674377243284,0.605845626926786));
#10228=CARTESIAN_POINT('Ctrl Pts',(1.09999997754868,-1.35674374570294,0.605845627052288));
#10229=CARTESIAN_POINT('Ctrl Pts',(1.09999999227748,-1.35627542940044,0.613744255356351));
#10230=CARTESIAN_POINT('Ctrl Pts',(1.1000044245081,-1.35483313756702,0.621542702113576));
#10231=CARTESIAN_POINT('Ctrl Pts',(1.10000632213307,-1.3525036790266,0.629082464357584));
#10232=CARTESIAN_POINT('Ctrl Pts',(1.1000073336739,-1.3512619466217,0.633101581650771));
#10233=CARTESIAN_POINT('Ctrl Pts',(1.10000777634458,-1.34976719347553,0.637047225321331));
#10234=CARTESIAN_POINT('Ctrl Pts',(1.10000752568741,-1.34802684471036,0.640893844816285));
#10235=CARTESIAN_POINT('Ctrl Pts',(1.10000705344834,-1.3447480208661,0.648140890909733));
#10236=CARTESIAN_POINT('Ctrl Pts',(1.10000374385205,-1.34063788586045,0.654954534019122));
#10237=CARTESIAN_POINT('Ctrl Pts',(1.10000230512149,-1.33576793982513,0.661175616324976));
#10238=CARTESIAN_POINT('Ctrl Pts',(1.10000200863552,-1.33476436716076,0.662457623989879));
#10239=CARTESIAN_POINT('Ctrl Pts',(1.10000181701501,-1.33372836971272,0.663714393476354));
#10240=CARTESIAN_POINT('Ctrl Pts',(1.10000180919237,-1.33266033853372,0.664944387472089));
#10241=CARTESIAN_POINT('Ctrl Pts',(1.10000179685332,-1.33097567746633,0.666884520904953));
#10242=CARTESIAN_POINT('Ctrl Pts',(1.10000223926429,-1.32921133126375,0.668758058859172));
#10243=CARTESIAN_POINT('Ctrl Pts',(1.10000288715521,-1.32737234926393,0.670562692084704));
#10244=CARTESIAN_POINT('Ctrl Pts',(1.10000489069569,-1.32168547392559,0.676143347135183));
#10245=CARTESIAN_POINT('Ctrl Pts',(1.10000845923633,-1.31535192007569,0.681005160308095));
#10246=CARTESIAN_POINT('Ctrl Pts',(1.1000097672184,-1.30853956043085,0.685101187995272));
#10247=CARTESIAN_POINT('Ctrl Pts',(1.10001062829021,-1.30405484229164,0.687797688271992));
#10248=CARTESIAN_POINT('Ctrl Pts',(1.10001067755751,-1.29936155475819,0.690161668140197));
#10249=CARTESIAN_POINT('Ctrl Pts',(1.10000992106221,-1.29450057597768,0.692169783635984));
#10250=CARTESIAN_POINT('Ctrl Pts',(1.10000876843985,-1.28709422081189,0.695229417764685));
#10251=CARTESIAN_POINT('Ctrl Pts',(1.100005676647,-1.27938091857402,0.69743146309387));
#10252=CARTESIAN_POINT('Ctrl Pts',(1.10000309801581,-1.2715114871423,0.698709794160748));
#10253=CARTESIAN_POINT('Ctrl Pts',(1.10000138449209,-1.26628217885177,0.699559256705032));
#10254=CARTESIAN_POINT('Ctrl Pts',(1.1,-1.26098326598685,0.700000000000001));
#10255=CARTESIAN_POINT('Ctrl Pts',(1.1,-1.25565664448621,0.7));
#10256=CARTESIAN_POINT('',(1.1,-1.39262953588351,0.));
#10257=CARTESIAN_POINT('Ctrl Pts',(1.1,-1.39262953588351,0.));
#10258=CARTESIAN_POINT('Ctrl Pts',(1.1,-1.38665944902278,0.100890429980357));
#10259=CARTESIAN_POINT('Ctrl Pts',(1.1,-1.38068638286488,0.201781712214768));
#10260=CARTESIAN_POINT('Ctrl Pts',(1.1,-1.36872453529477,0.403729561179669));
#10261=CARTESIAN_POINT('Ctrl Pts',(1.10000000000005,-1.3627356212621,0.504788200493074));
#10262=CARTESIAN_POINT('Ctrl Pts',(1.10000000000005,-1.35674377243284,0.605845626926786));
#10263=CARTESIAN_POINT('',(1.1,-1.44962962962963,0.));
#10264=CARTESIAN_POINT('Origin',(0.199725906950915,-1.4,-0.0104671912485888));
#10265=CARTESIAN_POINT('',(0.200274469199584,1.15262458915154,1.38777878078145E-17));
#10266=CARTESIAN_POINT('',(0.200274469199585,-0.7,0.));
#10267=CARTESIAN_POINT('',(0.231993417893744,1.12115139781563,0.605233595624295));
#10268=CARTESIAN_POINT('Ctrl Pts',(0.200274469199584,1.15262458915154,-5.50774703622636E-17));
#10269=CARTESIAN_POINT('Ctrl Pts',(0.210847451072758,1.1421331482829,0.201744512318911));
#10270=CARTESIAN_POINT('Ctrl Pts',(0.221420433966108,1.13164208276446,0.403489044103923));
#10271=CARTESIAN_POINT('Ctrl Pts',(0.231993417893744,1.12115139781563,0.605233595624295));
#10272=CARTESIAN_POINT('',(0.231993417893744,-1.12115139781563,0.605233595624295));
#10273=CARTESIAN_POINT('',(0.231993417893744,-0.7,0.605233595624295));
#10274=CARTESIAN_POINT('',(0.200274469199584,-1.15262458915154,1.38777878078145E-17));
#10275=CARTESIAN_POINT('Ctrl Pts',(0.231993417893744,-1.12115139781563,
0.605233595624295));
#10276=CARTESIAN_POINT('Ctrl Pts',(0.221420433966108,-1.13164208276446,
0.403489044103923));
#10277=CARTESIAN_POINT('Ctrl Pts',(0.210847451072758,-1.1421331482829,0.201744512318911));
#10278=CARTESIAN_POINT('Ctrl Pts',(0.200274469199584,-1.15262458915154,
-6.67868538251071E-17));
#10279=CARTESIAN_POINT('',(0.200274469199585,-0.7,0.));
#10280=CARTESIAN_POINT('Origin',(6.07974599480623,0.,0.));
#10281=CARTESIAN_POINT('Ctrl Pts',(8.1,-1.69866351109718,4.37041895728907E-16));
#10282=CARTESIAN_POINT('Ctrl Pts',(8.9524267631348,-1.65897367198627,1.20944032620455E-7));
#10283=CARTESIAN_POINT('Ctrl Pts',(9.80407798130771,-1.59837060538327,2.76830114922109E-8));
#10284=CARTESIAN_POINT('Ctrl Pts',(10.6537697771985,-1.52488560579501,1.03413542584124E-8));
#10285=CARTESIAN_POINT('Ctrl Pts',(10.8359404901627,-1.50913069933138,6.62336842220622E-9));
#10286=CARTESIAN_POINT('Ctrl Pts',(11.0180211259896,-1.49278349820154,3.93228299510406E-9));
#10287=CARTESIAN_POINT('Ctrl Pts',(11.2000000002909,-1.47592264092474,-3.0227174540096E-11));
#10288=CARTESIAN_POINT('Ctrl Pts',(11.2000000002909,1.47592264092474,-3.02272213335841E-11));
#10289=CARTESIAN_POINT('Ctrl Pts',(10.4240589919717,1.54781576943643,1.68591524001238E-8));
#10290=CARTESIAN_POINT('Ctrl Pts',(9.64626799696257,1.61037563220813,6.17878738288937E-8));
#10291=CARTESIAN_POINT('Ctrl Pts',(8.86753211358286,1.65747704847969,5.27022751808308E-8));
#10292=CARTESIAN_POINT('Ctrl Pts',(8.61177933690776,1.67294611604661,4.97183789310355E-8));
#10293=CARTESIAN_POINT('Ctrl Pts',(8.35592462822135,1.68674740550612,3.63007687033005E-8));
#10294=CARTESIAN_POINT('Ctrl Pts',(8.1,1.69866351109718,3.71000138306103E-16));
#10295=CARTESIAN_POINT('',(7.9,1.70758761671949,0.));
#10296=CARTESIAN_POINT('',(7.9,1.7737037037037,0.));
#10297=CARTESIAN_POINT('Ctrl Pts',(7.90000000036908,1.70758761645525,-3.06814577203155E-11));
#10298=CARTESIAN_POINT('Ctrl Pts',(7.26247716501442,1.73478515342832,3.65175246633048E-8));
#10299=CARTESIAN_POINT('Ctrl Pts',(6.624575449312,1.74993328406844,-3.04558542439636E-7));
#10300=CARTESIAN_POINT('Ctrl Pts',(5.98677261990733,1.74972113442148,-3.1918790057331E-7));
#10301=CARTESIAN_POINT('Ctrl Pts',(5.35540610719671,1.74951112565922,-3.33669628155763E-7));
#10302=CARTESIAN_POINT('Ctrl Pts',(4.72663057529054,1.73425216511322,1.21151810208783E-7));
#10303=CARTESIAN_POINT('Ctrl Pts',(4.10000000045307,1.7011388979176,-4.27317258673188E-11));
#10304=CARTESIAN_POINT('',(3.9,1.68995649764597,0.));
#10305=CARTESIAN_POINT('',(3.9,1.7662962962963,0.));
#10306=CARTESIAN_POINT('Ctrl Pts',(3.9,1.68995649764597,-1.6113354923472E-17));
#10307=CARTESIAN_POINT('Ctrl Pts',(2.96252047830716,1.63464572816558,-1.61179993858831E-17));
#10308=CARTESIAN_POINT('Ctrl Pts',(2.02971500398675,1.53866944530133,-1.61823222708931E-17));
#10309=CARTESIAN_POINT('Ctrl Pts',(1.1,1.39262953588351,-1.60717230190728E-17));
#10310=CARTESIAN_POINT('',(0.9,1.3604297237941,0.));
#10311=CARTESIAN_POINT('',(0.9,1.44962962962963,0.));
#10312=CARTESIAN_POINT('',(0.28146619846596,1.25073018526678,0.));
#10313=CARTESIAN_POINT('Ctrl Pts',(0.899999999999963,1.36042972379409,2.53412200078296E-14));
#10314=CARTESIAN_POINT('Ctrl Pts',(0.693681964344164,1.32640030945436,-1.68820282978727E-7));
#10315=CARTESIAN_POINT('Ctrl Pts',(0.487510176034459,1.28986876146525,1.95094241611213E-11));
#10316=CARTESIAN_POINT('Ctrl Pts',(0.281466198465954,1.25073018526678,9.09211941846344E-16));
#10317=CARTESIAN_POINT('Ctrl Pts',(0.28146619846596,1.25073018526678,4.90059381963448E-17));
#10318=CARTESIAN_POINT('Ctrl Pts',(0.273672142824666,1.24924968434803,-1.60851827685828E-11));
#10319=CARTESIAN_POINT('Ctrl Pts',(0.266112037439191,1.2468180315926,-2.29735811958388E-6));
#10320=CARTESIAN_POINT('Ctrl Pts',(0.258922416881026,1.24354471831116,-3.39045428380668E-6));
#10321=CARTESIAN_POINT('Ctrl Pts',(0.254316658841251,1.24144779416325,-4.09070493067818E-6));
#10322=CARTESIAN_POINT('Ctrl Pts',(0.249862973385875,1.23900427835211,-4.3601744978078E-6));
#10323=CARTESIAN_POINT('Ctrl Pts',(0.245601965247185,1.23623285256398,-4.0505643599354E-6));
#10324=CARTESIAN_POINT('Ctrl Pts',(0.238945660500109,1.23190348870705,-3.5669089987193E-6));
#10325=CARTESIAN_POINT('Ctrl Pts',(0.232836306411817,1.22682685988243,-1.47564048465526E-6));
#10326=CARTESIAN_POINT('Ctrl Pts',(0.227416445112993,1.2210931256102,-3.43092614100725E-7));
#10327=CARTESIAN_POINT('Ctrl Pts',(0.225957664245637,1.21954986437275,-3.82620891408318E-8));
#10328=CARTESIAN_POINT('Ctrl Pts',(0.224549002474426,1.21795876469157,1.76022586487844E-7));
#10329=CARTESIAN_POINT('Ctrl Pts',(0.223193686986583,1.21632111005909,2.01577349231486E-7));
#10330=CARTESIAN_POINT('Ctrl Pts',(0.221344954485829,1.21408724984631,2.36435595047204E-7));
#10331=CARTESIAN_POINT('Ctrl Pts',(0.219595448227346,1.21176677459781,-7.7718209010198E-8));
#10332=CARTESIAN_POINT('Ctrl Pts',(0.217948412504407,1.20936721934621,-5.08402878561E-7));
#10333=CARTESIAN_POINT('Ctrl Pts',(0.213467776427723,1.20283941082417,-1.68004793834142E-6));
#10334=CARTESIAN_POINT('Ctrl Pts',(0.20978887558685,1.19579640990262,-3.43350901357988E-6));
#10335=CARTESIAN_POINT('Ctrl Pts',(0.206958221875648,1.18840352636746,-3.67425174897535E-6));
#10336=CARTESIAN_POINT('Ctrl Pts',(0.206193447398199,1.18640614723908,-3.7392946395744E-6));
#10337=CARTESIAN_POINT('Ctrl Pts',(0.205490847532167,1.18438308363371,-3.7149036306613E-6));
#10338=CARTESIAN_POINT('Ctrl Pts',(0.204851940804359,1.18233735619935,-3.6037364623937E-6));
#10339=CARTESIAN_POINT('Ctrl Pts',(0.202492508448082,1.17478264548698,-3.19320484275276E-6));
#10340=CARTESIAN_POINT('Ctrl Pts',(0.201019195184615,1.16698811697394,-1.36638523817118E-6));
#10341=CARTESIAN_POINT('Ctrl Pts',(0.200491965466086,1.15911075533121,-4.28455138775697E-7));
#10342=CARTESIAN_POINT('Ctrl Pts',(0.200347608840846,1.15695391685535,-1.71647870329038E-7));
#10343=CARTESIAN_POINT('Ctrl Pts',(0.200274469313241,1.15479080601565,-7.49035961899928E-12));
#10344=CARTESIAN_POINT('Ctrl Pts',(0.200274469199584,1.15262458915154,9.10729824887824E-18));
#10345=CARTESIAN_POINT('',(2.01407162049393E-18,1.15316892111334,2.77409355997279E-17));
#10346=CARTESIAN_POINT('',(0.,-1.4,0.));
#10347=CARTESIAN_POINT('',(0.243580684154574,1.44748675362873,2.77555756156289E-17));
#10348=CARTESIAN_POINT('Ctrl Pts',(0.243580684154575,1.44748675362873,-1.56125112837913E-16));
#10349=CARTESIAN_POINT('Ctrl Pts',(0.226022619058538,1.44415189332774,-6.74769223000006E-12));
#10350=CARTESIAN_POINT('Ctrl Pts',(0.208837776424359,1.43922483814223,-1.83343972289099E-6));
#10351=CARTESIAN_POINT('Ctrl Pts',(0.192216855517481,1.43283671850359,-2.37047811876899E-6));
#10352=CARTESIAN_POINT('Ctrl Pts',(0.175448307189507,1.42639185943196,-2.91228650265529E-6));
#10353=CARTESIAN_POINT('Ctrl Pts',(0.15925228528901,1.41845922211561,-2.09168970691363E-6));
#10354=CARTESIAN_POINT('Ctrl Pts',(0.143842215871583,1.4091253227419,-1.20497646612983E-7));
#10355=CARTESIAN_POINT('Ctrl Pts',(0.141154971457358,1.40749765525544,2.23243494969264E-7));
#10356=CARTESIAN_POINT('Ctrl Pts',(0.138491701959641,1.40582727297256,5.92673833856784E-7));
#10357=CARTESIAN_POINT('Ctrl Pts',(0.135853645420207,1.40411450883245,9.74556207071009E-7));
#10358=CARTESIAN_POINT('Ctrl Pts',(0.120686164410185,1.39426698768136,3.17018528370531E-6));
#10359=CARTESIAN_POINT('Ctrl Pts',(0.106484701177391,1.38310949089167,6.09567884445769E-6));
#10360=CARTESIAN_POINT('Ctrl Pts',(0.0934509959242968,1.37075049507673,
5.10227143121889E-6));
#10361=CARTESIAN_POINT('Ctrl Pts',(0.0918301157095608,1.36921352217444,
4.97873062758527E-6));
#10362=CARTESIAN_POINT('Ctrl Pts',(0.0902273306836925,1.36765791150105,
4.78983320752683E-6));
#10363=CARTESIAN_POINT('Ctrl Pts',(0.0886430622088043,1.36608382581751,
4.52250464763623E-6));
#10364=CARTESIAN_POINT('Ctrl Pts',(0.0755027622673366,1.35302798437193,
2.30521792157715E-6));
#10365=CARTESIAN_POINT('Ctrl Pts',(0.0636322991078783,1.33870385142449,
-4.95851449924696E-6));
#10366=CARTESIAN_POINT('Ctrl Pts',(0.0531272107863483,1.3233265665666,-1.07771754856876E-5));
#10367=CARTESIAN_POINT('Ctrl Pts',(0.0429100363670196,1.3083707283404,-1.64363639061758E-5));
#10368=CARTESIAN_POINT('Ctrl Pts',(0.0340657397255946,1.29253754778979,
-2.07072841115287E-5));
#10369=CARTESIAN_POINT('Ctrl Pts',(0.026663056477648,1.27603964904139,-2.15377272154938E-5));
#10370=CARTESIAN_POINT('Ctrl Pts',(0.0217318501145713,1.26504977678014,
-2.20909166714363E-5));
#10371=CARTESIAN_POINT('Ctrl Pts',(0.0174411483101006,1.25376411673155,
-2.12025196266096E-5));
#10372=CARTESIAN_POINT('Ctrl Pts',(0.01382286588119,1.24224013948332,-1.91534441809703E-5));
#10373=CARTESIAN_POINT('Ctrl Pts',(0.00842668188255806,1.22505366970124,
-1.60975223868617E-5));
#10374=CARTESIAN_POINT('Ctrl Pts',(0.00456091079961661,1.20745571355567,
-1.03588883906395E-5));
#10375=CARTESIAN_POINT('Ctrl Pts',(0.0023097402764219,1.18964331095195,
-5.71664032024866E-6));
#10376=CARTESIAN_POINT('Ctrl Pts',(0.00078319128522165,1.17756448131848,
-2.56866950429304E-6));
#10377=CARTESIAN_POINT('Ctrl Pts',(2.50028438421117E-9,1.16538650529032,
-1.91718613723104E-10));
#10378=CARTESIAN_POINT('Ctrl Pts',(-1.21430643318376E-17,1.15316892111333,
5.20417042793042E-18));
#10379=CARTESIAN_POINT('',(11.7295909468525,1.62672708026858,5.55111512312578E-17));
#10380=CARTESIAN_POINT('Ctrl Pts',(0.243580684154574,1.44748675362873,0.));
#10381=CARTESIAN_POINT('Ctrl Pts',(4.07225077172054,2.17467835246083,0.));
#10382=CARTESIAN_POINT('Ctrl Pts',(7.90092085928651,2.00057770191527,0.));
#10383=CARTESIAN_POINT('Ctrl Pts',(11.7295909468525,1.62672708026858,0.));
#10384=CARTESIAN_POINT('',(12.,1.32855945177638,-4.17473993839455E-17));
#10385=CARTESIAN_POINT('Ctrl Pts',(12.,1.32855945177638,2.42861286636753E-16));
#10386=CARTESIAN_POINT('Ctrl Pts',(11.9999999991614,1.34640852075174,-1.28298622986823E-11));
#10387=CARTESIAN_POINT('Ctrl Pts',(11.9983618543561,1.36418409382152,-2.22383001277967E-6));
#10388=CARTESIAN_POINT('Ctrl Pts',(11.9951861391139,1.38167870884165,-3.43465861540838E-6));
#10389=CARTESIAN_POINT('Ctrl Pts',(11.9919727904737,1.39938064150867,-4.65983598400874E-6));
#10390=CARTESIAN_POINT('Ctrl Pts',(11.9871848331028,1.41679645887758,-4.78742071954366E-6));
#10391=CARTESIAN_POINT('Ctrl Pts',(11.9808755917115,1.43370272794343,-3.5739118077222E-6));
#10392=CARTESIAN_POINT('Ctrl Pts',(11.9797611226834,1.43668906371449,-3.35955670324834E-6));
#10393=CARTESIAN_POINT('Ctrl Pts',(11.9785990681726,1.43965944485564,-3.11247275469786E-6));
#10394=CARTESIAN_POINT('Ctrl Pts',(11.9773895732386,1.44261255525912,-2.84353511336506E-6));
#10395=CARTESIAN_POINT('Ctrl Pts',(11.9705369081732,1.45934406518776,-1.31980853313606E-6));
#10396=CARTESIAN_POINT('Ctrl Pts',(11.9622259501015,1.47537448669426,1.24030492427686E-6));
#10397=CARTESIAN_POINT('Ctrl Pts',(11.9525330320198,1.49048867890869,8.79804099270529E-7));
#10398=CARTESIAN_POINT('Ctrl Pts',(11.9492586078121,1.49559449703792,7.58021100761347E-7));
#10399=CARTESIAN_POINT('Ctrl Pts',(11.9458260650319,1.50059560584699,2.73671093112169E-7));
#10400=CARTESIAN_POINT('Ctrl Pts',(11.9422371454499,1.50548309160802,-8.21070286398525E-7));
#10401=CARTESIAN_POINT('Ctrl Pts',(11.9335276940755,1.51734385321214,-3.47774636801117E-6));
#10402=CARTESIAN_POINT('Ctrl Pts',(11.923898315087,1.52853671512454,-9.61160164537397E-6));
#10403=CARTESIAN_POINT('Ctrl Pts',(11.9134480753511,1.53899918600446,-1.54908303532852E-5));
#10404=CARTESIAN_POINT('Ctrl Pts',(11.9006414429521,1.55182080751067,-2.26957483986032E-5));
#10405=CARTESIAN_POINT('Ctrl Pts',(11.8867118754531,1.56343792791748,-2.93307907620841E-5));
#10406=CARTESIAN_POINT('Ctrl Pts',(11.8718669715436,1.57375979462261,-3.2097080434168E-5));
#10407=CARTESIAN_POINT('Ctrl Pts',(11.8583226919989,1.58317731924447,-3.46210038525051E-5));
#10408=CARTESIAN_POINT('Ctrl Pts',(11.84401509256,1.59151672629289,-3.39892197405707E-5));
#10409=CARTESIAN_POINT('Ctrl Pts',(11.8290799708805,1.59867837245092,-3.04453078860132E-5));
#10410=CARTESIAN_POINT('Ctrl Pts',(11.8128282236205,1.60647136308226,-2.65889777530425E-5));
#10411=CARTESIAN_POINT('Ctrl Pts',(11.7959622791259,1.61280865470064,-1.93051308245346E-5));
#10412=CARTESIAN_POINT('Ctrl Pts',(11.7786680578171,1.61758555622507,-1.24065785496921E-5));
#10413=CARTESIAN_POINT('Ctrl Pts',(11.7626326571209,1.62201475420184,-6.0101616208217E-6));
#10414=CARTESIAN_POINT('Ctrl Pts',(11.7462278952123,1.62510256303752,-1.15598952599692E-10));
#10415=CARTESIAN_POINT('Ctrl Pts',(11.7295909468525,1.62672708026857,-1.01481323344643E-16));
#10416=CARTESIAN_POINT('',(12.,-1.32855945177638,-2.7831599589297E-17));
#10417=CARTESIAN_POINT('',(12.,1.6,0.));
#10418=CARTESIAN_POINT('',(11.7295909468525,-1.62672708026858,-2.77555756156289E-17));
#10419=CARTESIAN_POINT('Ctrl Pts',(11.7295909468525,-1.62672708026858,2.76688394418301E-16));
#10420=CARTESIAN_POINT('Ctrl Pts',(11.7473502233519,-1.62499297457843,3.63491969896433E-13));
#10421=CARTESIAN_POINT('Ctrl Pts',(11.7648769397846,-1.62163540491215,-2.46542030701863E-6));
#10422=CARTESIAN_POINT('Ctrl Pts',(11.7819744899096,-1.61677476461769,-3.87870576098494E-6));
#10423=CARTESIAN_POINT('Ctrl Pts',(11.799277951102,-1.61185558613358,-5.30901184740094E-6));
#10424=CARTESIAN_POINT('Ctrl Pts',(11.8161433440738,-1.60539638769883,-5.61072687595782E-6));
#10425=CARTESIAN_POINT('Ctrl Pts',(11.8323535184498,-1.59747214364331,-4.43708131311936E-6));
#10426=CARTESIAN_POINT('Ctrl Pts',(11.8351986841263,-1.59608130189932,-4.23108623901291E-6));
#10427=CARTESIAN_POINT('Ctrl Pts',(11.8380235988884,-1.59464521634493,-3.98890160078043E-6));
#10428=CARTESIAN_POINT('Ctrl Pts',(11.8408269920241,-1.59316415515964,-3.72087260345577E-6));
#10429=CARTESIAN_POINT('Ctrl Pts',(11.8568148563263,-1.58471760338924,-2.19229240409177E-6));
#10430=CARTESIAN_POINT('Ctrl Pts',(11.8719627312575,-1.57488689795395,5.08047814114288E-7));
#10431=CARTESIAN_POINT('Ctrl Pts',(11.8860639991294,-1.56376935451958,3.7910357452838E-7));
#10432=CARTESIAN_POINT('Ctrl Pts',(11.8908390360804,-1.5600046802233,3.35439876042474E-7));
#10433=CARTESIAN_POINT('Ctrl Pts',(11.8954938739134,-1.55609205312677,-6.31409548673105E-8));
#10434=CARTESIAN_POINT('Ctrl Pts',(11.9000197537765,-1.55203410647271,-1.07033715310124E-6));
#10435=CARTESIAN_POINT('Ctrl Pts',(11.9109521284419,-1.54223203603875,-3.50324446252274E-6));
#10436=CARTESIAN_POINT('Ctrl Pts',(11.9211333865357,-1.53158293117673,-9.37257606292525E-6));
#10437=CARTESIAN_POINT('Ctrl Pts',(11.9305114837192,-1.52019095639426,-1.50133174764804E-5));
#10438=CARTESIAN_POINT('Ctrl Pts',(11.9420285825687,-1.50620064502377,-2.19406264148308E-5));
#10439=CARTESIAN_POINT('Ctrl Pts',(11.9522379825693,-1.49120969914507,-2.8349487615449E-5));
#10440=CARTESIAN_POINT('Ctrl Pts',(11.9610699533786,-1.47543375940277,-3.10096306454085E-5));
#10441=CARTESIAN_POINT('Ctrl Pts',(11.9691383866925,-1.46102167397773,-3.34398002084833E-5));
#10442=CARTESIAN_POINT('Ctrl Pts',(11.976057247492,-1.44595309822982,-3.28127654573608E-5));
#10443=CARTESIAN_POINT('Ctrl Pts',(11.9817405815488,-1.43037347552767,-2.93737351251587E-5));
#10444=CARTESIAN_POINT('Ctrl Pts',(11.9879190063177,-1.41343666945002,-2.56351214921306E-5));
#10445=CARTESIAN_POINT('Ctrl Pts',(11.9925890154887,-1.39602986621001,-1.86015881889918E-5));
#10446=CARTESIAN_POINT('Ctrl Pts',(11.9956646601292,-1.37834843064327,-1.1951505214167E-5));
#10447=CARTESIAN_POINT('Ctrl Pts',(11.9985188379205,-1.36194017591583,-5.78027239782095E-6));
#10448=CARTESIAN_POINT('Ctrl Pts',(11.9999999979315,-1.34529424449622,-1.63143103698095E-10));
#10449=CARTESIAN_POINT('Ctrl Pts',(12.,-1.32855945177638,6.07153216591882E-17));
#10450=CARTESIAN_POINT('',(0.243580684154574,-1.44748675362873,-2.77555756156289E-17));
#10451=CARTESIAN_POINT('Ctrl Pts',(11.7295909468525,-1.62672708026858,0.));
#10452=CARTESIAN_POINT('Ctrl Pts',(7.90092085928651,-2.00057770191527,0.));
#10453=CARTESIAN_POINT('Ctrl Pts',(4.07225077172054,-2.17467835246083,0.));
#10454=CARTESIAN_POINT('Ctrl Pts',(0.243580684154574,-1.44748675362873,
0.));
#10455=CARTESIAN_POINT('',(-2.01407162049393E-18,-1.15316892111334,-2.77409355997279E-17));
#10456=CARTESIAN_POINT('Ctrl Pts',(-1.45716771982052E-16,-1.15316892111333,
-8.67361737988404E-17));
#10457=CARTESIAN_POINT('Ctrl Pts',(1.25998894435939E-9,-1.17105087373522,
-1.90287520688926E-11));
#10458=CARTESIAN_POINT('Ctrl Pts',(0.00163339464743996,-1.18886359576077,
-1.42965894531121E-6));
#10459=CARTESIAN_POINT('Ctrl Pts',(0.00480727841906161,-1.20639511031145,
-1.64093682142839E-6));
#10460=CARTESIAN_POINT('Ctrl Pts',(0.00800796397580062,-1.22407466931478,
-1.8539988284852E-6));
#10461=CARTESIAN_POINT('Ctrl Pts',(0.0127756311263789,-1.24146980201313,
-7.66483898132055E-7));
#10462=CARTESIAN_POINT('Ctrl Pts',(0.0190655400899108,-1.25835467436912,
1.24978183846727E-6));
#10463=CARTESIAN_POINT('Ctrl Pts',(0.0201762582672253,-1.26133632875492,
1.60582880463507E-6));
#10464=CARTESIAN_POINT('Ctrl Pts',(0.0213345630164365,-1.2643020159517,
1.98173645466097E-6));
#10465=CARTESIAN_POINT('Ctrl Pts',(0.022540357064946,-1.26725040777374,
2.36324320385681E-6));
#10466=CARTESIAN_POINT('Ctrl Pts',(0.0293845669280623,-1.28398578013164,
4.5287143794027E-6));
#10467=CARTESIAN_POINT('Ctrl Pts',(0.0376942987862453,-1.30001720705818,
7.20349268724091E-6));
#10468=CARTESIAN_POINT('Ctrl Pts',(0.0474014865253391,-1.31512615530125,
5.82569015349308E-6));
#10469=CARTESIAN_POINT('Ctrl Pts',(0.0485928463173857,-1.31698047129067,
5.65659292531477E-6));
#10470=CARTESIAN_POINT('Ctrl Pts',(0.049805315173965,-1.3188208685659,5.4220814195758E-6));
#10471=CARTESIAN_POINT('Ctrl Pts',(0.0510388164126442,-1.32064691964073,
5.10992468070797E-6));
#10472=CARTESIAN_POINT('Ctrl Pts',(0.0614399911345998,-1.33604461498541,
2.47774509321499E-6));
#10473=CARTESIAN_POINT('Ctrl Pts',(0.0733332132114129,-1.35042574344132,
-5.3152380038924E-6));
#10474=CARTESIAN_POINT('Ctrl Pts',(0.0865238753361435,-1.36365441213776,
-1.1550981620978E-5));
#10475=CARTESIAN_POINT('Ctrl Pts',(0.0993129767592984,-1.37648036310613,
-1.75968917362996E-5));
#10476=CARTESIAN_POINT('Ctrl Pts',(0.113220041589059,-1.38812080263946,
-2.21381304374214E-5));
#10477=CARTESIAN_POINT('Ctrl Pts',(0.128049501721596,-1.3984678073416,-2.30260298918279E-5));
#10478=CARTESIAN_POINT('Ctrl Pts',(0.137898881094142,-1.40534004502052,
-2.36157518704412E-5));
#10479=CARTESIAN_POINT('Ctrl Pts',(0.148156110210342,-1.41164106947418,
-2.26770903305374E-5));
#10480=CARTESIAN_POINT('Ctrl Pts',(0.158771208267938,-1.41732893485082,
-2.05010084084185E-5));
#10481=CARTESIAN_POINT('Ctrl Pts',(0.174640735071984,-1.42583226958806,
-1.72477751171679E-5));
#10482=CARTESIAN_POINT('Ctrl Pts',(0.191199787345415,-1.4329086754137,-1.11085100333009E-5));
#10483=CARTESIAN_POINT('Ctrl Pts',(0.208270835533445,-1.43843835369108,
-6.12965879291162E-6));
#10484=CARTESIAN_POINT('Ctrl Pts',(0.219822542278978,-1.44218019901621,
-2.76054936125183E-6));
#10485=CARTESIAN_POINT('Ctrl Pts',(0.231609382520684,-1.4452130041726,-1.10646384277296E-10));
#10486=CARTESIAN_POINT('Ctrl Pts',(0.243580684154575,-1.44748675362873,
-8.67361737988404E-18));
#10487=CARTESIAN_POINT('',(0.,-1.4,0.));
#10488=CARTESIAN_POINT('',(0.28146619846596,-1.25073018526678,-1.38777878078145E-17));
#10489=CARTESIAN_POINT('Ctrl Pts',(0.200274469199584,-1.15262458915154,
-4.38017677684144E-17));
#10490=CARTESIAN_POINT('Ctrl Pts',(0.200274469606231,-1.16056122076396,
-2.67994619525583E-11));
#10491=CARTESIAN_POINT('Ctrl Pts',(0.201251993787099,-1.16844573575355,
-2.06906772440415E-6));
#10492=CARTESIAN_POINT('Ctrl Pts',(0.203125250303271,-1.17612349127761,
-3.03593176598444E-6));
#10493=CARTESIAN_POINT('Ctrl Pts',(0.204328175564463,-1.18105381768481,
-3.65681052429326E-6));
#10494=CARTESIAN_POINT('Ctrl Pts',(0.205901645655995,-1.18589907428975,
-3.87486521964464E-6));
#10495=CARTESIAN_POINT('Ctrl Pts',(0.207834893326199,-1.19061551412018,
-3.56660141708203E-6));
#10496=CARTESIAN_POINT('Ctrl Pts',(0.210845733886816,-1.19796089907112,
-3.08651126907409E-6));
#10497=CARTESIAN_POINT('Ctrl Pts',(0.214691665920849,-1.20490884791767,
-1.13290501265697E-6));
#10498=CARTESIAN_POINT('Ctrl Pts',(0.219311372289421,-1.21130241743461,
-1.88024479619773E-7));
#10499=CARTESIAN_POINT('Ctrl Pts',(0.220549822002528,-1.21301640393121,
6.52788543367939E-8));
#10500=CARTESIAN_POINT('Ctrl Pts',(0.22184414018537,-1.21469042595737,2.26073670777299E-7));
#10501=CARTESIAN_POINT('Ctrl Pts',(0.223193686901845,-1.21632111014354,
1.99977909429435E-7));
#10502=CARTESIAN_POINT('Ctrl Pts',(0.225054776233359,-1.21856990146355,
1.63990609064731E-7));
#10503=CARTESIAN_POINT('Ctrl Pts',(0.227020882846909,-1.2207363067163,-2.2494482424301E-7));
#10504=CARTESIAN_POINT('Ctrl Pts',(0.229085096241527,-1.22281561536867,
-7.25033596408456E-7));
#10505=CARTESIAN_POINT('Ctrl Pts',(0.234663732853057,-1.22843504764494,
-2.07654770860772E-6));
#10506=CARTESIAN_POINT('Ctrl Pts',(0.240898147116973,-1.23336261820331,
-3.93931381885212E-6));
#10507=CARTESIAN_POINT('Ctrl Pts',(0.247634917667946,-1.2375211924479,-4.15647360184107E-6));
#10508=CARTESIAN_POINT('Ctrl Pts',(0.24944409362824,-1.23863798757926,-4.21479238469909E-6));
#10509=CARTESIAN_POINT('Ctrl Pts',(0.251289686356224,-1.23969909864123,
-4.17584617698396E-6));
#10510=CARTESIAN_POINT('Ctrl Pts',(0.253169062337335,-1.24070249413235,
-4.04352721072409E-6));
#10511=CARTESIAN_POINT('Ctrl Pts',(0.260147540238377,-1.24442829106235,
-3.55220190316667E-6));
#10512=CARTESIAN_POINT('Ctrl Pts',(0.267526846148503,-1.24732811138375,
-1.51439637010182E-6));
#10513=CARTESIAN_POINT('Ctrl Pts',(0.275164162321015,-1.24931347733136,
-4.73394739174148E-7));
#10514=CARTESIAN_POINT('Ctrl Pts',(0.277246452424842,-1.24985478107889,
-1.89568936341825E-7));
#10515=CARTESIAN_POINT('Ctrl Pts',(0.27934803608603,-1.25032783487679,-4.20368826828312E-12));
#10516=CARTESIAN_POINT('Ctrl Pts',(0.28146619846596,-1.25073018526678,1.2793585635329E-17));
#10517=CARTESIAN_POINT('',(0.9,-1.3604297237941,0.));
#10518=CARTESIAN_POINT('Ctrl Pts',(0.281466198465954,-1.25073018526678,
9.63150999927498E-16));
#10519=CARTESIAN_POINT('Ctrl Pts',(0.487510152792939,-1.28986875705046,
1.95065110193295E-11));
#10520=CARTESIAN_POINT('Ctrl Pts',(0.693681940810289,-1.32640030557063,
-1.68784634270162E-7));
#10521=CARTESIAN_POINT('Ctrl Pts',(0.899999999999961,-1.36042972379409,
2.52314774976951E-14));
#10522=CARTESIAN_POINT('',(0.9,1.44962962962963,0.));
#10523=CARTESIAN_POINT('',(3.9,-1.68995649764597,0.));
#10524=CARTESIAN_POINT('Ctrl Pts',(1.1,-1.39262953588351,-2.05019623674552E-17));
#10525=CARTESIAN_POINT('Ctrl Pts',(2.02971449277185,-1.53866936499954,-2.04062575199768E-17));
#10526=CARTESIAN_POINT('Ctrl Pts',(2.96251993741879,-1.63464569625347,-2.05230086706555E-17));
#10527=CARTESIAN_POINT('Ctrl Pts',(3.9,-1.68995649764597,-2.05203881127908E-17));
#10528=CARTESIAN_POINT('',(3.9,1.7662962962963,0.));
#10529=CARTESIAN_POINT('',(7.9,-1.70758761671949,0.));
#10530=CARTESIAN_POINT('Ctrl Pts',(4.10000000045307,-1.7011388979176,-4.27317380631109E-11));
#10531=CARTESIAN_POINT('Ctrl Pts',(4.72643887491804,-1.7342420350347,1.20853286712337E-7));
#10532=CARTESIAN_POINT('Ctrl Pts',(5.35502164560988,-1.74950180199062,-3.33551248611792E-7));
#10533=CARTESIAN_POINT('Ctrl Pts',(5.98619394951577,-1.74972093772735,-3.1920111515717E-7));
#10534=CARTESIAN_POINT('Ctrl Pts',(6.62418968669829,-1.74994244248134,-3.0469584628258E-7));
#10535=CARTESIAN_POINT('Ctrl Pts',(7.26228442347589,-1.73479337602516,3.6583895104054E-8));
#10536=CARTESIAN_POINT('Ctrl Pts',(7.90000000036908,-1.70758761645525,-3.06816097140251E-11));
#10537=CARTESIAN_POINT('',(7.9,1.7737037037037,0.));
#10538=CARTESIAN_POINT('',(11.4,-1.45718524058191,0.));
#10539=CARTESIAN_POINT('',(11.7095901160181,-1.42740242188993,1.38777878078145E-17));
#10540=CARTESIAN_POINT('Ctrl Pts',(11.4000000008084,-1.45718524050535,1.02728155843002E-16));
#10541=CARTESIAN_POINT('Ctrl Pts',(11.5032315878449,-1.44740895658952,-1.62414911853346E-10));
#10542=CARTESIAN_POINT('Ctrl Pts',(11.6064290066394,-1.43747657129068,3.17212713797596E-13));
#10543=CARTESIAN_POINT('Ctrl Pts',(11.7095901160181,-1.42740242188993,-1.31135713082882E-16));
#10544=CARTESIAN_POINT('',(11.7997255308004,-1.32801330383774,0.));
#10545=CARTESIAN_POINT('Ctrl Pts',(11.7095901160181,-1.42740242188993,-9.19403442267708E-17));
#10546=CARTESIAN_POINT('Ctrl Pts',(11.7174875668098,-1.42663119997609,-1.06723531187443E-12));
#10547=CARTESIAN_POINT('Ctrl Pts',(11.7252481284326,-1.42489860698852,-1.31351091787008E-6));
#10548=CARTESIAN_POINT('Ctrl Pts',(11.7327147629935,-1.4222933789697,-1.57347087725304E-6));
#10549=CARTESIAN_POINT('Ctrl Pts',(11.7375034508718,-1.42062252930751,-1.7401948673154E-6));
#10550=CARTESIAN_POINT('Ctrl Pts',(11.742171336984,-1.41859157258352,-1.52962160850981E-6));
#10551=CARTESIAN_POINT('Ctrl Pts',(11.7466731630754,-1.4162133745499,-1.06822103866601E-6));
#10552=CARTESIAN_POINT('Ctrl Pts',(11.7538080604269,-1.41244419322064,-3.36952074275293E-7));
#10553=CARTESIAN_POINT('Ctrl Pts',(11.7604421378066,-1.40785009750528,1.23525126371337E-6));
#10554=CARTESIAN_POINT('Ctrl Pts',(11.7664060685299,-1.40250292630552,-7.85770423176645E-8));
#10555=CARTESIAN_POINT('Ctrl Pts',(11.7700505374369,-1.39923534992309,-8.81437879006801E-7));
#10556=CARTESIAN_POINT('Ctrl Pts',(11.7734443324447,-1.39568546479044,-2.84121358692309E-6));
#10557=CARTESIAN_POINT('Ctrl Pts',(11.7765701913309,-1.39188797822873,-4.73246891796253E-6));
#10558=CARTESIAN_POINT('Ctrl Pts',(11.7816218974528,-1.38575085342217,-7.78893003218221E-6));
#10559=CARTESIAN_POINT('Ctrl Pts',(11.7859196635778,-1.3790373064984,-1.04294718165207E-5));
#10560=CARTESIAN_POINT('Ctrl Pts',(11.7894058487846,-1.37190723377291,-1.0649753115785E-5));
#10561=CARTESIAN_POINT('Ctrl Pts',(11.7909886780302,-1.36866997385604,-1.07497672177443E-5));
#10562=CARTESIAN_POINT('Ctrl Pts',(11.7924036476919,-1.36534638272796,-1.04045251440782E-5));
#10563=CARTESIAN_POINT('Ctrl Pts',(11.7936422141268,-1.36194984358789,-9.67400732978531E-6));
#10564=CARTESIAN_POINT('Ctrl Pts',(11.7963517531347,-1.35451943450186,-8.0758964348484E-6));
#10565=CARTESIAN_POINT('Ctrl Pts',(11.7981920551596,-1.34681816044402,-4.45435127417515E-6));
#10566=CARTESIAN_POINT('Ctrl Pts',(11.7990923524223,-1.33899256731255,-1.99131993767782E-6));
#10567=CARTESIAN_POINT('Ctrl Pts',(11.7995108157868,-1.33535518645399,-8.46488755312323E-7));
#10568=CARTESIAN_POINT('Ctrl Pts',(11.7997255306472,-1.33169069466208,-1.20180646731727E-11));
#10569=CARTESIAN_POINT('Ctrl Pts',(11.7997255308004,-1.32801330383774,1.56125112837913E-17));
#10570=CARTESIAN_POINT('',(11.7997255308004,1.32801330383774,-1.38777878078145E-17));
#10571=CARTESIAN_POINT('',(11.7997255308004,0.8,0.));
#10572=CARTESIAN_POINT('',(11.7095901160181,1.42740242188993,1.38777878078145E-17));
#10573=CARTESIAN_POINT('Ctrl Pts',(11.7997255308004,1.32801330383774,3.29597460435593E-17));
#10574=CARTESIAN_POINT('Ctrl Pts',(11.7997255306701,1.33594993357028,-3.19998942079111E-12));
#10575=CARTESIAN_POINT('Ctrl Pts',(11.7987557313351,1.34384388324515,-1.1738056914779E-6));
#10576=CARTESIAN_POINT('Ctrl Pts',(11.7968890528831,1.35153020534854,-1.35082478761126E-6));
#10577=CARTESIAN_POINT('Ctrl Pts',(11.7956902940742,1.35646627043222,-1.46450435604653E-6));
#10578=CARTESIAN_POINT('Ctrl Pts',(11.7941204989552,1.36131691981906,-1.21679535622301E-6));
#10579=CARTESIAN_POINT('Ctrl Pts',(11.7921880664813,1.36603565236267,-7.51718013047842E-7));
#10580=CARTESIAN_POINT('Ctrl Pts',(11.7891321441143,1.37349779167052,-1.62510435539431E-8));
#10581=CARTESIAN_POINT('Ctrl Pts',(11.7852081688769,1.38054242009704,1.47305143123643E-6));
#10582=CARTESIAN_POINT('Ctrl Pts',(11.7804707482717,1.38699431162271,4.31295153147674E-8));
#10583=CARTESIAN_POINT('Ctrl Pts',(11.7775673564694,1.39094843993989,-8.33217322910001E-7));
#10584=CARTESIAN_POINT('Ctrl Pts',(11.774357304366,1.39467961749964,-2.88177890715362E-6));
#10585=CARTESIAN_POINT('Ctrl Pts',(11.7708736118052,1.39816709864095,-4.85419454747415E-6));
#10586=CARTESIAN_POINT('Ctrl Pts',(11.7652557092992,1.40379111072049,-8.03496856102318E-6));
#10587=CARTESIAN_POINT('Ctrl Pts',(11.7589908599241,1.40872063947841,-1.07717451179728E-5));
#10588=CARTESIAN_POINT('Ctrl Pts',(11.7522324303862,1.41288246393566,-1.10093962897399E-5));
#10589=CARTESIAN_POINT('Ctrl Pts',(11.7491699691574,1.41476832010531,-1.11170836593312E-5));
#10590=CARTESIAN_POINT('Ctrl Pts',(11.7460056456443,1.41649603445901,-1.07652933077188E-5));
#10591=CARTESIAN_POINT('Ctrl Pts',(11.7427518690514,1.41805582819498,-1.00150721194158E-5));
#10592=CARTESIAN_POINT('Ctrl Pts',(11.7356218627913,1.421473806899,-8.37111113549047E-6));
#10593=CARTESIAN_POINT('Ctrl Pts',(11.7281378774234,1.42405291512428,-4.62166314666036E-6));
#10594=CARTESIAN_POINT('Ctrl Pts',(11.7204387731059,1.42570834923663,-2.06587013620581E-6));
#10595=CARTESIAN_POINT('Ctrl Pts',(11.7168648812537,1.42647679479109,-8.79481766934018E-7));
#10596=CARTESIAN_POINT('Ctrl Pts',(11.7132443218769,1.42704557200794,-8.45784208685192E-12));
#10597=CARTESIAN_POINT('Ctrl Pts',(11.7095901160181,1.42740242188993,2.53703308361608E-17));
#10598=CARTESIAN_POINT('',(11.4,1.45718524058191,0.));
#10599=CARTESIAN_POINT('Ctrl Pts',(11.7095901160181,1.42740242188993,-2.09644042577228E-16));
#10600=CARTESIAN_POINT('Ctrl Pts',(11.6064290073882,1.43747657121756,3.16925904777201E-13));
#10601=CARTESIAN_POINT('Ctrl Pts',(11.5032315885351,1.44740895652415,-1.62368751268212E-10));
#10602=CARTESIAN_POINT('Ctrl Pts',(11.4000000008083,1.45718524050537,-7.57963810214684E-17));
#10603=CARTESIAN_POINT('',(11.4,-1.53779953703704,0.));
#10604=CARTESIAN_POINT('Origin',(10.,0.,0.));
#10605=CARTESIAN_POINT('',(9.6,-4.89858719658942E-17,0.7));
#10606=CARTESIAN_POINT('Origin',(10.,0.,0.7));
#10607=CARTESIAN_POINT('',(9.6,-4.89858719658942E-17,0.));
#10608=CARTESIAN_POINT('Origin',(2.,0.,0.));
#10609=CARTESIAN_POINT('',(1.6,-4.89858719658941E-17,0.7));
#10610=CARTESIAN_POINT('Origin',(2.,0.,0.7));
#10611=CARTESIAN_POINT('',(1.6,-4.89858719658941E-17,0.));
#10612=CARTESIAN_POINT('Origin',(11.4,-1.53779953703704,0.));
#10613=CARTESIAN_POINT('',(11.4,-1.4227102204299,0.605660349289938));
#10614=CARTESIAN_POINT('Ctrl Pts',(11.4,-1.45718524058191,0.));
#10615=CARTESIAN_POINT('Ctrl Pts',(11.4,-1.45144762186897,0.100853500740053));
#10616=CARTESIAN_POINT('Ctrl Pts',(11.4,-1.44570843451869,0.201707502489292));
#10617=CARTESIAN_POINT('Ctrl Pts',(11.4,-1.43421679834229,0.403593890565801));
#10618=CARTESIAN_POINT('Ctrl Pts',(11.4,-1.42846427656079,0.504627461196798));
#10619=CARTESIAN_POINT('Ctrl Pts',(11.4,-1.4227102204299,0.605660349289938));
#10620=CARTESIAN_POINT('',(11.4,1.4227102204299,0.605660349289938));
#10621=CARTESIAN_POINT('Ctrl Pts',(11.4,1.4227102204299,0.605660349289938));
#10622=CARTESIAN_POINT('Ctrl Pts',(11.4,1.42846501637408,0.504614471147338));
#10623=CARTESIAN_POINT('Ctrl Pts',(11.4,1.43421827757761,0.403567910233218));
#10624=CARTESIAN_POINT('Ctrl Pts',(11.4,1.44570991295315,0.201681522149997));
#10625=CARTESIAN_POINT('Ctrl Pts',(11.4,1.45144836088146,0.100840510682596));
#10626=CARTESIAN_POINT('Ctrl Pts',(11.4,1.45718524058191,0.));
#10627=CARTESIAN_POINT('',(11.4,1.32241589772268,0.7));
#10628=CARTESIAN_POINT('Ctrl Pts',(11.3999999999682,1.32241589773435,0.7));
#10629=CARTESIAN_POINT('Ctrl Pts',(11.4000000023735,1.33035873561384,0.69999999792071));
#10630=CARTESIAN_POINT('Ctrl Pts',(11.3999980827719,1.33823923135401,0.699006238562837));
#10631=CARTESIAN_POINT('Ctrl Pts',(11.3999964146773,1.34591623266897,0.697118452648154));
#10632=CARTESIAN_POINT('Ctrl Pts',(11.3999954805754,1.35021521026861,0.696061327733467));
#10633=CARTESIAN_POINT('Ctrl Pts',(11.3999946303028,1.35445042327231,0.694722827332644));
#10634=CARTESIAN_POINT('Ctrl Pts',(11.3999940855437,1.35859537550353,0.6931136259882));
#10635=CARTESIAN_POINT('Ctrl Pts',(11.3999931076272,1.36603612757745,0.690224891070856));
#10636=CARTESIAN_POINT('Ctrl Pts',(11.3999932937992,1.3731074395729,0.686497549823264));
#10637=CARTESIAN_POINT('Ctrl Pts',(11.3999945206258,1.37966241828116,0.682010734965951));
#10638=CARTESIAN_POINT('Ctrl Pts',(11.3999951957832,1.38326980879772,0.679541513617388));
#10639=CARTESIAN_POINT('Ctrl Pts',(11.399996159718,1.38672054258633,0.67684140394947));
#10640=CARTESIAN_POINT('Ctrl Pts',(11.3999970106794,1.38998612808193,0.67391813047908));
#10641=CARTESIAN_POINT('Ctrl Pts',(11.399997834674,1.39314822810011,0.671087494715186));
#10642=CARTESIAN_POINT('Ctrl Pts',(11.3999985616145,1.39611771109305,0.668064564866167));
#10643=CARTESIAN_POINT('Ctrl Pts',(11.3999985600482,1.39887227052748,0.664860274403491));
#10644=CARTESIAN_POINT('Ctrl Pts',(11.3999985571253,1.40401282028653,0.65888043807832));
#10645=CARTESIAN_POINT('Ctrl Pts',(11.3999962993541,1.40840780441339,0.652270325570232));
#10646=CARTESIAN_POINT('Ctrl Pts',(11.399995545677,1.411994629421,0.6451936465425));
#10647=CARTESIAN_POINT('Ctrl Pts',(11.3999954685939,1.41236147527551,0.644469872631166));
#10648=CARTESIAN_POINT('Ctrl Pts',(11.3999954033687,1.41271982702329,0.643741199273148));
#10649=CARTESIAN_POINT('Ctrl Pts',(11.399995351278,1.41306958904162,0.643007791034547));
#10650=CARTESIAN_POINT('Ctrl Pts',(11.3999948427782,1.41648390439843,0.635848388696429));
#10651=CARTESIAN_POINT('Ctrl Pts',(11.3999960181446,1.41904356023948,0.628323447569199));
#10652=CARTESIAN_POINT('Ctrl Pts',(11.3999977140636,1.42069349507095,0.620600117586001));
#10653=CARTESIAN_POINT('Ctrl Pts',(11.3999987928026,1.4217429844709,0.615687467222433));
#10654=CARTESIAN_POINT('Ctrl Pts',(11.4,1.42242354791745,0.610693903223035));
#10655=CARTESIAN_POINT('Ctrl Pts',(11.4,1.42271022042989,0.605660349289938));
#10656=CARTESIAN_POINT('',(11.4,-1.32241589772233,0.7));
#10657=CARTESIAN_POINT('',(11.4,-0.768899768518519,0.7));
#10658=CARTESIAN_POINT('Ctrl Pts',(11.4,-1.4227102204299,0.605660349289938));
#10659=CARTESIAN_POINT('Ctrl Pts',(11.4,-1.42225988230954,0.613567634148305));
#10660=CARTESIAN_POINT('Ctrl Pts',(11.399997277834,-1.42084002197897,0.621378952482038));
#10661=CARTESIAN_POINT('Ctrl Pts',(11.3999960666067,-1.41853584574224,0.62893480307212));
#10662=CARTESIAN_POINT('Ctrl Pts',(11.3999954054252,-1.41727804822547,0.633059370437125));
#10663=CARTESIAN_POINT('Ctrl Pts',(11.399995101512,-1.41575577202439,0.637107840337094));
#10664=CARTESIAN_POINT('Ctrl Pts',(11.3999952458732,-1.4139766528271,0.641052464558972));
#10665=CARTESIAN_POINT('Ctrl Pts',(11.3999955106959,-1.41071295596475,0.648288661951321));
#10666=CARTESIAN_POINT('Ctrl Pts',(11.3999975070228,-1.40662392062869,0.655096264526915));
#10667=CARTESIAN_POINT('Ctrl Pts',(11.3999983091255,-1.40177626405188,0.661313589686923));
#10668=CARTESIAN_POINT('Ctrl Pts',(11.3999984645713,-1.40083679843637,0.66251849418371));
#10669=CARTESIAN_POINT('Ctrl Pts',(11.3999985618942,-1.3998687022723,0.663701157110503));
#10670=CARTESIAN_POINT('Ctrl Pts',(11.3999985615247,-1.39887227038638,0.664860274403572));
#10671=CARTESIAN_POINT('Ctrl Pts',(11.3999985608543,-1.39706426040285,0.666963474499402));
#10672=CARTESIAN_POINT('Ctrl Pts',(11.3999982409398,-1.39516298427334,0.668989190735049));
#10673=CARTESIAN_POINT('Ctrl Pts',(11.3999977953094,-1.39317470503404,0.670934323115149));
#10674=CARTESIAN_POINT('Ctrl Pts',(11.3999965209597,-1.38748891009577,0.67649673287249));
#10675=CARTESIAN_POINT('Ctrl Pts',(11.3999944455422,-1.38115857071774,0.681340422576046));
#10676=CARTESIAN_POINT('Ctrl Pts',(11.3999937508435,-1.37434881732181,0.685413525744465));
#10677=CARTESIAN_POINT('Ctrl Pts',(11.3999933041982,-1.36997059693002,0.688032261301096));
#10678=CARTESIAN_POINT('Ctrl Pts',(11.3999933336943,-1.3653932120823,0.69033179581025));
#10679=CARTESIAN_POINT('Ctrl Pts',(11.399993839827,-1.36065445462682,0.69228884175444));
#10680=CARTESIAN_POINT('Ctrl Pts',(11.3999946245508,-1.35330733883187,0.695323106179894));
#10681=CARTESIAN_POINT('Ctrl Pts',(11.3999965692242,-1.34565642326237,0.69750197024776));
#10682=CARTESIAN_POINT('Ctrl Pts',(11.3999981510416,-1.33784990929195,0.698756936804364));
#10683=CARTESIAN_POINT('Ctrl Pts',(11.399999182603,-1.33275899381189,0.699575346749464));
#10684=CARTESIAN_POINT('Ctrl Pts',(11.4000000015384,-1.32760128986121,0.699999998642559));
#10685=CARTESIAN_POINT('Ctrl Pts',(11.3999999999682,-1.32241589773435,0.7));
#10686=CARTESIAN_POINT('Ctrl Pts',(11.227882892666,-1.47337141465794,-0.000640335460849732));
#10687=CARTESIAN_POINT('Ctrl Pts',(11.218588765022,-1.46278323638644,0.201451598614313));
#10688=CARTESIAN_POINT('Ctrl Pts',(11.2092944683555,-1.45219508216535,0.40354352620373));
#10689=CARTESIAN_POINT('Ctrl Pts',(11.2000000000001,-1.44160695250309,0.60563544721184));
#10690=CARTESIAN_POINT('Ctrl Pts',(10.1843397214697,-1.57034855377304,-0.000384310983874139));
#10691=CARTESIAN_POINT('Ctrl Pts',(10.1768953195658,-1.55975965902304,0.201708049868595));
#10692=CARTESIAN_POINT('Ctrl Pts',(10.1694507716805,-1.54917076711515,0.403800406245857));
#10693=CARTESIAN_POINT('Ctrl Pts',(10.1620060668616,-1.53858190981164,0.605892758286982));
#10694=CARTESIAN_POINT('Ctrl Pts',(9.14170648965309,-1.65016851777514,-0.000148134864058495));
#10695=CARTESIAN_POINT('Ctrl Pts',(9.13611341817177,-1.63957870617509,0.201944615677573));
#10696=CARTESIAN_POINT('Ctrl Pts',(9.13052023035058,-1.6289888900612,0.404037363603497));
#10697=CARTESIAN_POINT('Ctrl Pts',(9.124926910836,-1.6183991014662,0.606130109186173));
#10698=CARTESIAN_POINT('Ctrl Pts',(8.1,-1.69866351109718,1.00613961606655E-16));
#10699=CARTESIAN_POINT('Ctrl Pts',(8.09625995443094,-1.68807302815665,0.202092993803311));
#10700=CARTESIAN_POINT('Ctrl Pts',(8.09251982249141,-1.67748255132318,0.404185986335255));
#10701=CARTESIAN_POINT('Ctrl Pts',(8.08877960280056,-1.66689208072706,0.606278977577217));
#10702=CARTESIAN_POINT('Ctrl Pts',(8.1,-1.66641703131627,0.605314487869832));
#10703=CARTESIAN_POINT('Ctrl Pts',(9.13548525483003,-1.617718421277,0.605389190939432));
#10704=CARTESIAN_POINT('Ctrl Pts',(10.168822041161,-1.53796707615457,0.605507632815633));
#10705=CARTESIAN_POINT('Ctrl Pts',(11.2000000000893,-1.44160695345912,0.605635447210802));
#10706=CARTESIAN_POINT('Ctrl Pts',(11.7095939787209,-1.42740645209206,-7.69249563980189E-5));
#10707=CARTESIAN_POINT('Ctrl Pts',(11.6994545874061,-1.41682738380082,0.201847033339061));
#10708=CARTESIAN_POINT('Ctrl Pts',(11.6893150192885,-1.40624834198077,0.403770984173611));
#10709=CARTESIAN_POINT('Ctrl Pts',(11.6791752715866,-1.39566932719028,0.605694927437301));
#10710=CARTESIAN_POINT('Ctrl Pts',(11.6063871276792,-1.43748358609578,-5.11721697277706E-5));
#10711=CARTESIAN_POINT('Ctrl Pts',(11.596430427176,-1.42690445239132,0.201872829148883));
#10712=CARTESIAN_POINT('Ctrl Pts',(11.5864735514701,-1.41632534465399,0.403796823219986));
#10713=CARTESIAN_POINT('Ctrl Pts',(11.5765164978042,-1.40574626343445,0.605720809936841));
#10714=CARTESIAN_POINT('Ctrl Pts',(11.5031891278894,-1.4474144288224,-2.55082377288765E-5));
#10715=CARTESIAN_POINT('Ctrl Pts',(11.4934151336386,-1.43683522760458,0.201898535909597));
#10716=CARTESIAN_POINT('Ctrl Pts',(11.4836409658656,-1.42625605183456,0.40382257302165));
#10717=CARTESIAN_POINT('Ctrl Pts',(11.4738666218385,-1.41567690205216,0.605746602994839));
#10718=CARTESIAN_POINT('Ctrl Pts',(11.4,-1.45718524058191,-5.20417042793042E-18));
#10719=CARTESIAN_POINT('Ctrl Pts',(11.3904087275488,-1.44660597001679,0.201924086674796));
#10720=CARTESIAN_POINT('Ctrl Pts',(11.3808172833376,-1.43602672436683,0.403848166524883));
#10721=CARTESIAN_POINT('Ctrl Pts',(11.3712256646606,-1.42544750415802,0.605772239449758));
#10722=CARTESIAN_POINT('',(11.6778970386953,-1.39579479040469,0.605695249702977));
#10723=CARTESIAN_POINT('Ctrl Pts',(11.4,-1.4227102204299,0.605660349289938));
#10724=CARTESIAN_POINT('Ctrl Pts',(11.4926474653491,-1.41386220753305,0.605671932550561));
#10725=CARTESIAN_POINT('Ctrl Pts',(11.585279512325,-1.40488700096013,0.605683574233495));
#10726=CARTESIAN_POINT('Ctrl Pts',(11.6778970386953,-1.39579479040469,0.605695249702977));
#10727=CARTESIAN_POINT('Ctrl Pts',(11.6778970386953,-1.39579479040469,0.605695249702977));
#10728=CARTESIAN_POINT('Ctrl Pts',(11.6884613130147,-1.40633044792991,0.403796817797553));
#10729=CARTESIAN_POINT('Ctrl Pts',(11.6990256725537,-1.41686632615463,0.201898401304098));
#10730=CARTESIAN_POINT('Ctrl Pts',(11.7095901160181,-1.42740242188993,5.19332840620557E-17));
#10731=CARTESIAN_POINT('Ctrl Pts',(11.2,-1.34133050917871,0.7));
#10732=CARTESIAN_POINT('Ctrl Pts',(10.1668086441106,-1.43797263608903,0.7));
#10733=CARTESIAN_POINT('Ctrl Pts',(9.13190264019122,-1.51792184128158,0.7));
#10734=CARTESIAN_POINT('Ctrl Pts',(8.09530923905977,-1.56666858280461,0.7));
#10735=CARTESIAN_POINT('Ctrl Pts',(11.2026864299662,-1.37005086445236,0.7));
#10736=CARTESIAN_POINT('Ctrl Pts',(10.1691860218014,-1.46674693471719,0.700000910790016));
#10737=CARTESIAN_POINT('Ctrl Pts',(9.13384227773975,-1.54675516497,0.699999464833944));
#10738=CARTESIAN_POINT('Ctrl Pts',(8.09666712422266,-1.59554384206015,0.700000000000001));
#10739=CARTESIAN_POINT('Ctrl Pts',(11.2073428085028,-1.4198317437391,0.676744232988519));
#10740=CARTESIAN_POINT('Ctrl Pts',(10.1733099382853,-1.51661799675652,0.676702307311825));
#10741=CARTESIAN_POINT('Ctrl Pts',(9.13719745543551,-1.59672983278297,0.676663906627884));
#10742=CARTESIAN_POINT('Ctrl Pts',(8.09902054834098,-1.64558911349573,0.676639354455264));
#10743=CARTESIAN_POINT('Ctrl Pts',(11.2091847227485,-1.43952346553595,0.627236497176141));
#10744=CARTESIAN_POINT('Ctrl Pts',(10.1749352046592,-1.53629892039422,0.62712791425818));
#10745=CARTESIAN_POINT('Ctrl Pts',(9.13852107143019,-1.61640633519008,0.627027713743691));
#10746=CARTESIAN_POINT('Ctrl Pts',(8.0999458765183,-1.66526610220338,0.626964226563296));
#10747=CARTESIAN_POINT('Ctrl Pts',(11.209298290232,-1.4407376041935,0.605636599993194));
#10748=CARTESIAN_POINT('Ctrl Pts',(10.1750338985877,-1.53748737250229,0.605508345221004));
#10749=CARTESIAN_POINT('Ctrl Pts',(9.13859765097935,-1.61757204607208,0.605389415477198));
#10750=CARTESIAN_POINT('Ctrl Pts',(8.1,-1.66641703131627,0.605314487869832));
#10751=CARTESIAN_POINT('Ctrl Pts',(11.2,-1.34133050917871,0.7));
#10752=CARTESIAN_POINT('Ctrl Pts',(10.16836710286,-1.43782686176815,0.7));
#10753=CARTESIAN_POINT('Ctrl Pts',(9.13502472651537,-1.51768061363633,0.7));
#10754=CARTESIAN_POINT('Ctrl Pts',(8.09999999865516,-1.56644778212326,0.7));
#10755=CARTESIAN_POINT('Ctrl Pts',(11.6681436286308,-1.2964346619681,0.7));
#10756=CARTESIAN_POINT('Ctrl Pts',(11.5756099286391,-1.3055179747114,0.7));
#10757=CARTESIAN_POINT('Ctrl Pts',(11.4830653488871,-1.31448403714215,0.7));
#10758=CARTESIAN_POINT('Ctrl Pts',(11.3905090053564,-1.32332268868375,0.7));
#10759=CARTESIAN_POINT('Ctrl Pts',(11.6709605510772,-1.32513126902304,0.700000000000001));
#10760=CARTESIAN_POINT('Ctrl Pts',(11.5784027531871,-1.33421922733773,0.700000082825348));
#10761=CARTESIAN_POINT('Ctrl Pts',(11.4858332859074,-1.34318985044544,0.699999917777441));
#10762=CARTESIAN_POINT('Ctrl Pts',(11.3932507170007,-1.35203326785046,0.7));
#10763=CARTESIAN_POINT('Ctrl Pts',(11.6758431636759,-1.37487151491717,0.67676311428296));
#10764=CARTESIAN_POINT('Ctrl Pts',(11.583243842395,-1.38396722707511,0.676759299309384));
#10765=CARTESIAN_POINT('Ctrl Pts',(11.4906306781253,-1.39294591144353,0.676755553516685));
#10766=CARTESIAN_POINT('Ctrl Pts',(11.3980029235659,-1.40179729139028,0.67675176769038));
#10767=CARTESIAN_POINT('Ctrl Pts',(11.6777767156198,-1.39456903283364,0.627286048421068));
#10768=CARTESIAN_POINT('Ctrl Pts',(11.5851604051362,-1.40366358810601,0.627276165220861));
#10769=CARTESIAN_POINT('Ctrl Pts',(11.4925297866457,-1.41264104586547,0.627266369072496));
#10770=CARTESIAN_POINT('Ctrl Pts',(11.3998836071583,-1.4214913811319,0.627256563056779));
#10771=CARTESIAN_POINT('Ctrl Pts',(11.6778970386953,-1.39579479040469,0.605695249702977));
#10772=CARTESIAN_POINT('Ctrl Pts',(11.585279512325,-1.40488700096013,0.605683574233495));
#10773=CARTESIAN_POINT('Ctrl Pts',(11.4926474653491,-1.41386220753305,0.605671932550561));
#10774=CARTESIAN_POINT('Ctrl Pts',(11.4,-1.4227102204299,0.605660349289938));
#10775=CARTESIAN_POINT('',(11.6681436286308,-1.2964346619681,0.7));
#10776=CARTESIAN_POINT('Ctrl Pts',(11.6681436286308,-1.2964346619681,0.7));
#10777=CARTESIAN_POINT('Ctrl Pts',(11.5787728332608,-1.30520749699507,0.7));
#10778=CARTESIAN_POINT('Ctrl Pts',(11.4893918891838,-1.31387096021207,0.7));
#10779=CARTESIAN_POINT('Ctrl Pts',(11.3999999999682,-1.32241589773435,0.7));
#10780=CARTESIAN_POINT('Origin',(11.6681436286308,-1.2964346619681,0.6));
#10781=CARTESIAN_POINT('Origin',(6.08012166120517,1.06778195214465E-16,
0.7));
#10782=CARTESIAN_POINT('Ctrl Pts',(8.0999999986552,1.56644778212326,0.7));
#10783=CARTESIAN_POINT('Ctrl Pts',(9.13502472651542,1.51768061363633,0.7));
#10784=CARTESIAN_POINT('Ctrl Pts',(10.16836710286,1.43782686176815,0.7));
#10785=CARTESIAN_POINT('Ctrl Pts',(11.2,1.34133050917871,0.7));
#10786=CARTESIAN_POINT('Origin',(6.08012166120517,1.06778195214465E-16,
0.7));
#10787=CARTESIAN_POINT('',(11.6681436286308,1.2964346619681,0.7));
#10788=CARTESIAN_POINT('Ctrl Pts',(11.3999999999682,1.32241589773435,0.7));
#10789=CARTESIAN_POINT('Ctrl Pts',(11.4893918891837,1.31387096021208,0.7));
#10790=CARTESIAN_POINT('Ctrl Pts',(11.5787728332608,1.30520749699508,0.7));
#10791=CARTESIAN_POINT('Ctrl Pts',(11.6681436286308,1.2964346619681,0.7));
#10792=CARTESIAN_POINT('',(11.6681436286308,0.8,0.7));
#10793=CARTESIAN_POINT('Ctrl Pts',(8.09530923905978,1.56666858280461,0.7));
#10794=CARTESIAN_POINT('Ctrl Pts',(9.13190264019124,1.51792184128158,0.7));
#10795=CARTESIAN_POINT('Ctrl Pts',(10.1668086441106,1.43797263608903,0.7));
#10796=CARTESIAN_POINT('Ctrl Pts',(11.2,1.34133050917871,0.7));
#10797=CARTESIAN_POINT('Ctrl Pts',(8.09666712422266,1.59554384206015,0.700000000000001));
#10798=CARTESIAN_POINT('Ctrl Pts',(9.13384227773977,1.54675516497,0.699999464833944));
#10799=CARTESIAN_POINT('Ctrl Pts',(10.1691860218013,1.46674693471719,0.700000910790016));
#10800=CARTESIAN_POINT('Ctrl Pts',(11.2026864299662,1.37005086445236,0.7));
#10801=CARTESIAN_POINT('Ctrl Pts',(8.09902054834099,1.64558911349573,0.676639354455264));
#10802=CARTESIAN_POINT('Ctrl Pts',(9.13719745543553,1.59672983278297,0.676663906627884));
#10803=CARTESIAN_POINT('Ctrl Pts',(10.1733099382853,1.51661799675652,0.676702307311825));
#10804=CARTESIAN_POINT('Ctrl Pts',(11.2073428085028,1.4198317437391,0.676744232988519));
#10805=CARTESIAN_POINT('Ctrl Pts',(8.0999458765183,1.66526610220338,0.626964226563296));
#10806=CARTESIAN_POINT('Ctrl Pts',(9.1385210714302,1.61640633519008,0.627027713743691));
#10807=CARTESIAN_POINT('Ctrl Pts',(10.1749352046592,1.53629892039423,0.62712791425818));
#10808=CARTESIAN_POINT('Ctrl Pts',(11.2091847227485,1.43952346553595,0.627236497176141));
#10809=CARTESIAN_POINT('Ctrl Pts',(8.1,1.66641703131627,0.605314487869832));
#10810=CARTESIAN_POINT('Ctrl Pts',(9.13859765097937,1.61757204607208,0.605389415477198));
#10811=CARTESIAN_POINT('Ctrl Pts',(10.1750338985877,1.53748737250229,0.605508345221004));
#10812=CARTESIAN_POINT('Ctrl Pts',(11.209298290232,1.4407376041935,0.605636599993194));
#10813=CARTESIAN_POINT('Ctrl Pts',(11.2000000000893,1.44160695345912,0.605635447210802));
#10814=CARTESIAN_POINT('Ctrl Pts',(10.168822041161,1.53796707615457,0.605507632815633));
#10815=CARTESIAN_POINT('Ctrl Pts',(9.13548525483005,1.617718421277,0.605389190939432));
#10816=CARTESIAN_POINT('Ctrl Pts',(8.1,1.66641703131627,0.605314487869832));
#10817=CARTESIAN_POINT('Ctrl Pts',(8.1,1.69866351109859,-2.6441702993818E-11));
#10818=CARTESIAN_POINT('Ctrl Pts',(8.09625995443078,1.68807302815759,0.202092993785684));
#10819=CARTESIAN_POINT('Ctrl Pts',(8.09251982249108,1.67748255132366,0.404185986326441));
#10820=CARTESIAN_POINT('Ctrl Pts',(8.08877960280008,1.66689208072708,0.606278977577217));
#10821=CARTESIAN_POINT('Ctrl Pts',(9.14170648965349,1.65016851777655,-0.00014813489050026));
#10822=CARTESIAN_POINT('Ctrl Pts',(9.13611341817193,1.63957870617604,0.201944615659945));
#10823=CARTESIAN_POINT('Ctrl Pts',(9.1305202303505,1.62898889006169,0.404037363594684));
#10824=CARTESIAN_POINT('Ctrl Pts',(9.12492691083567,1.61839910146622,0.606130109186173));
#10825=CARTESIAN_POINT('Ctrl Pts',(10.1843397214705,1.57034855377444,-0.000384311010315772));
#10826=CARTESIAN_POINT('Ctrl Pts',(10.1768953195662,1.55975965902398,0.201708049850968));
#10827=CARTESIAN_POINT('Ctrl Pts',(10.1694507716807,1.54917076711562,0.403800406237042));
#10828=CARTESIAN_POINT('Ctrl Pts',(10.1620060668615,1.53858190981166,0.605892758286982));
#10829=CARTESIAN_POINT('Ctrl Pts',(11.2278828926672,1.47337141465933,-0.000640335487291374));
#10830=CARTESIAN_POINT('Ctrl Pts',(11.2185887650228,1.46278323638736,0.201451598596686));
#10831=CARTESIAN_POINT('Ctrl Pts',(11.2092944683559,1.45219508216582,0.403543526194916));
#10832=CARTESIAN_POINT('Ctrl Pts',(11.2000000000001,1.44160695250309,0.60563544721184));
#10833=CARTESIAN_POINT('Ctrl Pts',(11.4,1.45718524058191,-1.37043154602168E-16));
#10834=CARTESIAN_POINT('Ctrl Pts',(11.3904087275488,1.44660597001679,0.201924086674796));
#10835=CARTESIAN_POINT('Ctrl Pts',(11.3808172833376,1.43602672436683,0.403848166524884));
#10836=CARTESIAN_POINT('Ctrl Pts',(11.3712256646606,1.42544750415802,0.605772239449759));
#10837=CARTESIAN_POINT('Ctrl Pts',(11.5031891278894,1.4474144288224,-2.55082377290153E-5));
#10838=CARTESIAN_POINT('Ctrl Pts',(11.4934151336386,1.43683522760458,0.201898535909598));
#10839=CARTESIAN_POINT('Ctrl Pts',(11.4836409658656,1.42625605183455,0.40382257302165));
#10840=CARTESIAN_POINT('Ctrl Pts',(11.4738666218385,1.41567690205216,0.605746602994839));
#10841=CARTESIAN_POINT('Ctrl Pts',(11.6063871276792,1.43748358609579,-5.1172169727805E-5));
#10842=CARTESIAN_POINT('Ctrl Pts',(11.596430427176,1.42690445239132,0.201872829148883));
#10843=CARTESIAN_POINT('Ctrl Pts',(11.5864735514701,1.41632534465399,0.403796823219986));
#10844=CARTESIAN_POINT('Ctrl Pts',(11.5765164978042,1.40574626343445,0.605720809936842));
#10845=CARTESIAN_POINT('Ctrl Pts',(11.7095939787209,1.42740645209206,-7.69249563980588E-5));
#10846=CARTESIAN_POINT('Ctrl Pts',(11.6994545874061,1.41682738380082,0.201847033339061));
#10847=CARTESIAN_POINT('Ctrl Pts',(11.6893150192885,1.40624834198077,0.403770984173611));
#10848=CARTESIAN_POINT('Ctrl Pts',(11.6791752715866,1.39566932719028,0.605694927437301));
#10849=CARTESIAN_POINT('',(11.6778970386953,1.39579479040469,0.605695249702977));
#10850=CARTESIAN_POINT('Ctrl Pts',(11.7095901160181,1.42740242188993,2.01986864734049E-16));
#10851=CARTESIAN_POINT('Ctrl Pts',(11.6990256725537,1.41686632615463,0.201898401304098));
#10852=CARTESIAN_POINT('Ctrl Pts',(11.6884613130147,1.40633044792991,0.403796817797553));
#10853=CARTESIAN_POINT('Ctrl Pts',(11.6778970386953,1.39579479040469,0.605695249702978));
#10854=CARTESIAN_POINT('Ctrl Pts',(11.6778970386953,1.39579479040469,0.605695249702977));
#10855=CARTESIAN_POINT('Ctrl Pts',(11.585279512325,1.40488700096013,0.605683574233495));
#10856=CARTESIAN_POINT('Ctrl Pts',(11.4926474653491,1.41386220753305,0.605671932550561));
#10857=CARTESIAN_POINT('Ctrl Pts',(11.4,1.4227102204299,0.605660349289938));
#10858=CARTESIAN_POINT('Origin',(7.9,1.7737037037037,0.));
#10859=CARTESIAN_POINT('',(7.9,-1.67543132363858,0.605300614462415));
#10860=CARTESIAN_POINT('Ctrl Pts',(7.9,-1.67543132363858,0.605300614462415));
#10861=CARTESIAN_POINT('Ctrl Pts',(7.9,-1.68078196203297,0.504592238472094));
#10862=CARTESIAN_POINT('Ctrl Pts',(7.9,-1.68613236521525,0.403883028813119));
#10863=CARTESIAN_POINT('Ctrl Pts',(7.9,-1.69685110017509,0.202116711316755));
#10864=CARTESIAN_POINT('Ctrl Pts',(7.9,-1.70221951791351,0.10105794916591));
#10865=CARTESIAN_POINT('Ctrl Pts',(7.9,-1.70758761671949,0.));
#10866=CARTESIAN_POINT('',(7.9,-1.57547905376932,0.7));
#10867=CARTESIAN_POINT('Ctrl Pts',(7.9,-1.57547905376882,0.7));
#10868=CARTESIAN_POINT('Ctrl Pts',(7.9,-1.58339333479856,0.700000000000001));
#10869=CARTESIAN_POINT('Ctrl Pts',(7.89999913038498,-1.59124411312484,0.699006032637452));
#10870=CARTESIAN_POINT('Ctrl Pts',(7.89999837104309,-1.59889106951376,0.697118831203047));
#10871=CARTESIAN_POINT('Ctrl Pts',(7.89999794343345,-1.6031973145812,0.696056087876834));
#10872=CARTESIAN_POINT('Ctrl Pts',(7.89999755365678,-1.60743898057435,0.694709047589066));
#10873=CARTESIAN_POINT('Ctrl Pts',(7.89999730661842,-1.61158931211603,0.693088720937666));
#10874=CARTESIAN_POINT('Ctrl Pts',(7.89999686465941,-1.6190143793929,0.690189908089508));
#10875=CARTESIAN_POINT('Ctrl Pts',(7.89999696143539,-1.626066934352,0.686450944759811));
#10876=CARTESIAN_POINT('Ctrl Pts',(7.89999752554231,-1.63260082031789,0.681953255064161));
#10877=CARTESIAN_POINT('Ctrl Pts',(7.89999783650325,-1.63620259020663,0.679473927540052));
#10878=CARTESIAN_POINT('Ctrl Pts',(7.89999827825103,-1.63964648551863,0.676763160200805));
#10879=CARTESIAN_POINT('Ctrl Pts',(7.89999867021687,-1.64290407802379,0.673829034208746));
#10880=CARTESIAN_POINT('Ctrl Pts',(7.89999905115172,-1.64606999298761,0.670977482527793));
#10881=CARTESIAN_POINT('Ctrl Pts',(7.89999938859403,-1.64904076201529,0.667932171841817));
#10882=CARTESIAN_POINT('Ctrl Pts',(7.89999938783828,-1.6517939440564,0.66470449824639));
#10883=CARTESIAN_POINT('Ctrl Pts',(7.89999938643498,-1.65690611124346,0.658711285012161));
#10884=CARTESIAN_POINT('Ctrl Pts',(7.89999834643869,-1.661271022418,0.652090721578155));
#10885=CARTESIAN_POINT('Ctrl Pts',(7.89999799057748,-1.66482884904143,0.645008203309728));
#10886=CARTESIAN_POINT('Ctrl Pts',(7.89999795399159,-1.66519462718329,0.644280053614395));
#10887=CARTESIAN_POINT('Ctrl Pts',(7.89999792287445,-1.66555183396469,0.643547001244109));
#10888=CARTESIAN_POINT('Ctrl Pts',(7.89999789784292,-1.66590037542058,0.642809214685104));
#10889=CARTESIAN_POINT('Ctrl Pts',(7.89999765441981,-1.66928982250308,0.635634491398386));
#10890=CARTESIAN_POINT('Ctrl Pts',(7.89999817709027,-1.67182454272713,0.628096763436417));
#10891=CARTESIAN_POINT('Ctrl Pts',(7.8999989464625,-1.67345106343068,0.620364350320046));
#10892=CARTESIAN_POINT('Ctrl Pts',(7.89999943944948,-1.67449328136075,0.615409688768565));
#10893=CARTESIAN_POINT('Ctrl Pts',(7.89999999630063,-1.67516175160204,0.610374426093907));
#10894=CARTESIAN_POINT('Ctrl Pts',(7.89999999769359,-1.67543132314592,0.605300614465834));
#10895=CARTESIAN_POINT('',(7.9,1.57547905376882,0.7));
#10896=CARTESIAN_POINT('',(7.9,0.886851851851852,0.7));
#10897=CARTESIAN_POINT('',(7.9,1.67543132363858,0.605300614462415));
#10898=CARTESIAN_POINT('Ctrl Pts',(7.89999999769359,1.67543132314592,0.605300614465834));
#10899=CARTESIAN_POINT('Ctrl Pts',(7.89999999552123,1.67501091691767,0.613213400729193));
#10900=CARTESIAN_POINT('Ctrl Pts',(7.89999875799714,1.67362284400845,0.621034919585595));
#10901=CARTESIAN_POINT('Ctrl Pts',(7.89999821041927,1.67135120200026,0.628604813990272));
#10902=CARTESIAN_POINT('Ctrl Pts',(7.89999790518813,1.67008494211401,0.632824428521627));
#10903=CARTESIAN_POINT('Ctrl Pts',(7.89999777089825,1.66854314417455,0.636965893954691));
#10904=CARTESIAN_POINT('Ctrl Pts',(7.89999784944871,1.66673368022774,0.640999456224326));
#10905=CARTESIAN_POINT('Ctrl Pts',(7.89999799035603,1.66348778281681,0.648235040746992));
#10906=CARTESIAN_POINT('Ctrl Pts',(7.8999989183875,1.65941887886545,0.655045206964536));
#10907=CARTESIAN_POINT('Ctrl Pts',(7.89999927807636,1.65459101651367,0.661266862646797));
#10908=CARTESIAN_POINT('Ctrl Pts',(7.89999934554656,1.65368540929837,0.662433916689859));
#10909=CARTESIAN_POINT('Ctrl Pts',(7.89999938740919,1.65275296801062,0.663580193269421));
#10910=CARTESIAN_POINT('Ctrl Pts',(7.89999938728957,1.65179394408007,0.664704498246374));
#10911=CARTESIAN_POINT('Ctrl Pts',(7.89999938705343,1.64990069294102,0.666924037937161));
#10912=CARTESIAN_POINT('Ctrl Pts',(7.89999922461202,1.64790387543569,0.669057997255949));
#10913=CARTESIAN_POINT('Ctrl Pts',(7.89999900301747,1.64581073954063,0.671102663899023));
#10914=CARTESIAN_POINT('Ctrl Pts',(7.89999840121276,1.64012621790684,0.676655553128015));
#10915=CARTESIAN_POINT('Ctrl Pts',(7.89999746538644,1.63379824275617,0.681490110487894));
#10916=CARTESIAN_POINT('Ctrl Pts',(7.89999715581736,1.6269906793715,0.685552192443336));
#10917=CARTESIAN_POINT('Ctrl Pts',(7.89999695885968,1.62265949106942,0.688136618155352));
#10918=CARTESIAN_POINT('Ctrl Pts',(7.89999697413705,1.61813320929371,0.690407672840119));
#10919=CARTESIAN_POINT('Ctrl Pts',(7.89999720528031,1.61344832872307,0.692342105328139));
#10920=CARTESIAN_POINT('Ctrl Pts',(7.89999756646959,1.60612763680413,0.69536488980882));
#10921=CARTESIAN_POINT('Ctrl Pts',(7.89999845750109,1.59850458633822,0.69753330980446));
#10922=CARTESIAN_POINT('Ctrl Pts',(7.89999917312139,1.59072625322659,0.698777780766876));
#10923=CARTESIAN_POINT('Ctrl Pts',(7.8999996358458,1.58569673594883,0.699582463224842));
#10924=CARTESIAN_POINT('Ctrl Pts',(7.9,1.58060170040825,0.7));
#10925=CARTESIAN_POINT('Ctrl Pts',(7.9,1.57547905376882,0.7));
#10926=CARTESIAN_POINT('Ctrl Pts',(7.9,1.70758761671949,0.));
#10927=CARTESIAN_POINT('Ctrl Pts',(7.9,1.70221949782947,0.101058327261027));
#10928=CARTESIAN_POINT('Ctrl Pts',(7.9,1.69685105999395,0.202117467714));
#10929=CARTESIAN_POINT('Ctrl Pts',(7.9,1.68613232500772,0.403883785628764));
#10930=CARTESIAN_POINT('Ctrl Pts',(7.9,1.6807819419292,0.504592616860323));
#10931=CARTESIAN_POINT('Ctrl Pts',(7.9,1.67543132363858,0.605300614462415));
#10932=CARTESIAN_POINT('Ctrl Pts',(7.91019312999368,-1.70715886092982,-0.000134090250286965));
#10933=CARTESIAN_POINT('Ctrl Pts',(7.90679525219671,-1.69658223918655,0.201692187253877));
#10934=CARTESIAN_POINT('Ctrl Pts',(7.90339729501941,-1.68600562260833,0.40351846369823));
#10935=CARTESIAN_POINT('Ctrl Pts',(7.89999925719352,-1.67542901130525,0.605344739067286));
#10936=CARTESIAN_POINT('Ctrl Pts',(6.63535348802246,-1.76179300886274,3.38453142643293E-5));
#10937=CARTESIAN_POINT('Ctrl Pts',(6.63422081661327,-1.7512156246026,0.201860399405878));
#10938=CARTESIAN_POINT('Ctrl Pts',(6.6330881724013,-1.74063821514668,0.403686949685767));
#10939=CARTESIAN_POINT('Ctrl Pts',(6.63195543348167,-1.7300608292057,0.605513504373875));
#10940=CARTESIAN_POINT('Ctrl Pts',(5.36191629096386,-1.76821426310706,6.25694230841134E-5));
#10941=CARTESIAN_POINT('Ctrl Pts',(5.36305144950513,-1.75763653444312,0.201889164820622));
#10942=CARTESIAN_POINT('Ctrl Pts',(5.36418670601529,-1.74705878452761,0.403715755186214));
#10943=CARTESIAN_POINT('Ctrl Pts',(5.36532191986746,-1.73648104871457,0.605542351516859));
#10944=CARTESIAN_POINT('Ctrl Pts',(4.08978435919194,-1.70060618495018,-0.000163379468877527));
#10945=CARTESIAN_POINT('Ctrl Pts',(4.09318947412453,-1.69002991101751,0.201662855819258));
#10946=CARTESIAN_POINT('Ctrl Pts',(4.09659468720556,-1.67945364498778,0.403489089874722));
#10947=CARTESIAN_POINT('Ctrl Pts',(4.1,-1.66887738702936,0.605315322680078));
#10948=CARTESIAN_POINT('Ctrl Pts',(4.10000000006189,-1.66887738587128,0.605315322687833));
#10949=CARTESIAN_POINT('Ctrl Pts',(5.36600428635239,-1.73653511802878,0.605201749988751));
#10950=CARTESIAN_POINT('Ctrl Pts',(6.63469107356441,-1.72995836404769,0.605216415547347));
#10951=CARTESIAN_POINT('Ctrl Pts',(7.89999999997453,-1.67543132304763,0.605300614465986));
#10952=CARTESIAN_POINT('Ctrl Pts',(7.9,-1.57547905376882,0.7));
#10953=CARTESIAN_POINT('Ctrl Pts',(6.63400208894818,-1.63014048526579,0.7));
#10954=CARTESIAN_POINT('Ctrl Pts',(5.36531976402288,-1.63670020240541,0.7));
#10955=CARTESIAN_POINT('Ctrl Pts',(4.09999999999999,-1.56887583540973,0.7));
#10956=CARTESIAN_POINT('Ctrl Pts',(7.9012470621039,-1.60436190544783,0.700000000000001));
#10957=CARTESIAN_POINT('Ctrl Pts',(6.6345175325877,-1.65907137725265,0.700000604190856));
#10958=CARTESIAN_POINT('Ctrl Pts',(5.36490325870521,-1.66564852467601,0.700000815814724));
#10959=CARTESIAN_POINT('Ctrl Pts',(4.09845273665223,-1.59774131518914,0.699999999999999));
#10960=CARTESIAN_POINT('Ctrl Pts',(7.90340849276168,-1.6544221878571,0.676636720659303));
#10961=CARTESIAN_POINT('Ctrl Pts',(6.63541917043928,-1.70921256696412,0.676609005714152));
#10962=CARTESIAN_POINT('Ctrl Pts',(5.36416860778507,-1.71581908642683,0.67660414986632));
#10963=CARTESIAN_POINT('Ctrl Pts',(4.09577098158984,-1.64777167791894,0.676641578059328));
#10964=CARTESIAN_POINT('Ctrl Pts',(7.90425799286387,-1.67409721877663,0.626952737571144));
#10965=CARTESIAN_POINT('Ctrl Pts',(6.63576820027036,-1.72888861107585,0.626881076846221));
#10966=CARTESIAN_POINT('Ctrl Pts',(5.36388821219926,-1.73550154452763,0.626868555890157));
#10967=CARTESIAN_POINT('Ctrl Pts',(4.09471668402893,-1.66744047248441,0.626965338598652));
#10968=CARTESIAN_POINT('Ctrl Pts',(7.90430757201307,-1.67524550738887,0.605300901379154));
#10969=CARTESIAN_POINT('Ctrl Pts',(6.63578978311492,-1.73002023206136,0.605216330280387));
#10970=CARTESIAN_POINT('Ctrl Pts',(5.3638700255334,-1.7366305488338,0.605201579557148));
#10971=CARTESIAN_POINT('Ctrl Pts',(4.09465499692593,-1.6685912965035,0.605315802949303));
#10972=CARTESIAN_POINT('Ctrl Pts',(7.9,-1.57547905376882,0.7));
#10973=CARTESIAN_POINT('Ctrl Pts',(6.63400208894818,-1.63014048526579,0.7));
#10974=CARTESIAN_POINT('Ctrl Pts',(5.36531976402288,-1.63670020240541,0.7));
#10975=CARTESIAN_POINT('Ctrl Pts',(4.09999999999999,-1.56887583540973,0.7));
#10976=CARTESIAN_POINT('Origin',(6.08012166120517,1.06778195214465E-16,
0.7));
#10977=CARTESIAN_POINT('Ctrl Pts',(4.1,1.56887583540973,0.7));
#10978=CARTESIAN_POINT('Ctrl Pts',(5.36531976402291,1.63670020240541,0.7));
#10979=CARTESIAN_POINT('Ctrl Pts',(6.63400208894819,1.63014048526579,0.7));
#10980=CARTESIAN_POINT('Ctrl Pts',(7.9,1.57547905376882,0.7));
#10981=CARTESIAN_POINT('Ctrl Pts',(4.1,1.56887583540973,0.7));
#10982=CARTESIAN_POINT('Ctrl Pts',(5.36531976402291,1.63670020240541,0.7));
#10983=CARTESIAN_POINT('Ctrl Pts',(6.63400208894819,1.63014048526579,0.7));
#10984=CARTESIAN_POINT('Ctrl Pts',(7.9,1.57547905376882,0.7));
#10985=CARTESIAN_POINT('Ctrl Pts',(4.09845273665224,1.59774131518914,0.699999999999999));
#10986=CARTESIAN_POINT('Ctrl Pts',(5.36490325870523,1.66564852467601,0.700000815814725));
#10987=CARTESIAN_POINT('Ctrl Pts',(6.6345175325877,1.65907137725265,0.700000604190856));
#10988=CARTESIAN_POINT('Ctrl Pts',(7.9012470621039,1.60436190544783,0.700000000000001));
#10989=CARTESIAN_POINT('Ctrl Pts',(4.09577098158985,1.64777167791894,0.676641578059328));
#10990=CARTESIAN_POINT('Ctrl Pts',(5.36416860778509,1.71581908642683,0.67660414986632));
#10991=CARTESIAN_POINT('Ctrl Pts',(6.6354191704393,1.70921256696412,0.676609005714152));
#10992=CARTESIAN_POINT('Ctrl Pts',(7.90340849276168,1.6544221878571,0.676636720659302));
#10993=CARTESIAN_POINT('Ctrl Pts',(4.09471668402895,1.66744047248441,0.626965338598652));
#10994=CARTESIAN_POINT('Ctrl Pts',(5.36388821219928,1.73550154452763,0.626868555890157));
#10995=CARTESIAN_POINT('Ctrl Pts',(6.63576820027036,1.72888861107585,0.626881076846221));
#10996=CARTESIAN_POINT('Ctrl Pts',(7.90425799286387,1.67409721877663,0.626952737571144));
#10997=CARTESIAN_POINT('Ctrl Pts',(4.09465499692594,1.6685912965035,0.605315802949303));
#10998=CARTESIAN_POINT('Ctrl Pts',(5.36387002553342,1.7366305488338,0.605201579557148));
#10999=CARTESIAN_POINT('Ctrl Pts',(6.63578978311492,1.73002023206136,0.605216330280387));
#11000=CARTESIAN_POINT('Ctrl Pts',(7.90430757201307,1.67524550738887,0.605300901379154));
#11001=CARTESIAN_POINT('Ctrl Pts',(7.89999999997454,1.67543132304763,0.605300614465986));
#11002=CARTESIAN_POINT('Ctrl Pts',(6.63469107356441,1.72995836404769,0.605216415547348));
#11003=CARTESIAN_POINT('Ctrl Pts',(5.36600428635241,1.73653511802878,0.605201749988751));
#11004=CARTESIAN_POINT('Ctrl Pts',(4.10000000006189,1.66887738587128,0.605315322687833));
#11005=CARTESIAN_POINT('Ctrl Pts',(4.08978435969213,1.70060618339657,-0.000163349821525811));
#11006=CARTESIAN_POINT('Ctrl Pts',(4.093189474458,1.69002990998177,0.201662875584159));
#11007=CARTESIAN_POINT('Ctrl Pts',(4.0965946873723,1.67945364446992,0.403489099757173));
#11008=CARTESIAN_POINT('Ctrl Pts',(4.1,1.66887738702936,0.605315322680078));
#11009=CARTESIAN_POINT('Ctrl Pts',(5.36191629113061,1.76821426155324,6.25990704884337E-5));
#11010=CARTESIAN_POINT('Ctrl Pts',(5.3630514496163,1.75763653340724,0.201889184585558));
#11011=CARTESIAN_POINT('Ctrl Pts',(5.36418670607087,1.74705878400967,0.403715765068683));
#11012=CARTESIAN_POINT('Ctrl Pts',(5.36532191986745,1.73648104871457,0.605542351516858));
#11013=CARTESIAN_POINT('Ctrl Pts',(6.63535348785608,1.76179300730897,3.38749616628245E-5));
#11014=CARTESIAN_POINT('Ctrl Pts',(6.63422081650235,1.75121562356675,0.20186041917081));
#11015=CARTESIAN_POINT('Ctrl Pts',(6.63308817234583,1.74063821462875,0.403686959568233));
#11016=CARTESIAN_POINT('Ctrl Pts',(6.63195543348166,1.7300608292057,0.605513504373875));
#11017=CARTESIAN_POINT('Ctrl Pts',(7.91019312949454,1.70715885937616,-0.000134060602928919));
#11018=CARTESIAN_POINT('Ctrl Pts',(7.90679525186394,1.69658223815078,0.201692207018782));
#11019=CARTESIAN_POINT('Ctrl Pts',(7.90339729485302,1.68600562209044,0.403518473580683));
#11020=CARTESIAN_POINT('Ctrl Pts',(7.89999925719352,1.67542901130525,0.605344739067286));
#11021=CARTESIAN_POINT('Origin',(3.9,1.7662962962963,0.));
#11022=CARTESIAN_POINT('',(3.9,-1.657567947596,0.605334330700044));
#11023=CARTESIAN_POINT('Ctrl Pts',(3.9,-1.657567947596,0.605334330700044));
#11024=CARTESIAN_POINT('Ctrl Pts',(3.9,-1.66295505583237,0.504667750148195));
#11025=CARTESIAN_POINT('Ctrl Pts',(3.9,-1.66834175427306,0.404000185805616));
#11026=CARTESIAN_POINT('Ctrl Pts',(3.9,-1.67913790341918,0.202222727053817));
#11027=CARTESIAN_POINT('Ctrl Pts',(3.9,-1.68454745406112,0.101110889248462));
#11028=CARTESIAN_POINT('Ctrl Pts',(3.9,-1.68995649764597,0.));
#11029=CARTESIAN_POINT('',(3.9,-1.55753217754889,0.7));
#11030=CARTESIAN_POINT('Ctrl Pts',(3.89999999700315,-1.55753217437,0.7));
#11031=CARTESIAN_POINT('Ctrl Pts',(3.89999999197785,-1.56545359401377,0.699999998841372));
#11032=CARTESIAN_POINT('Ctrl Pts',(3.90000117861029,-1.57331197233837,0.699006163267487));
#11033=CARTESIAN_POINT('Ctrl Pts',(3.90000221019459,-1.58096665047841,0.697118921400131));
#11034=CARTESIAN_POINT('Ctrl Pts',(3.90000279139136,-1.58527931230009,0.696055645348449));
#11035=CARTESIAN_POINT('Ctrl Pts',(3.90000331912093,-1.58952737074567,0.694707745526415));
#11036=CARTESIAN_POINT('Ctrl Pts',(3.90000364796674,-1.59368396010392,0.693086194530447));
#11037=CARTESIAN_POINT('Ctrl Pts',(3.90000423564848,-1.60111221870485,0.690188313817561));
#11038=CARTESIAN_POINT('Ctrl Pts',(3.90000407815102,-1.60816848972648,0.686450841450731));
#11039=CARTESIAN_POINT('Ctrl Pts',(3.9000032813392,-1.6147063365644,0.681954558458482));
#11040=CARTESIAN_POINT('Ctrl Pts',(3.90000284137901,-1.61831621321653,0.679471932695374));
#11041=CARTESIAN_POINT('Ctrl Pts',(3.90000222202081,-1.62176776859012,0.67675708350434));
#11042=CARTESIAN_POINT('Ctrl Pts',(3.9000016760669,-1.6250323621476,0.673818036286869));
#11043=CARTESIAN_POINT('Ctrl Pts',(3.90000114791654,-1.62819049732732,0.670974831382826));
#11044=CARTESIAN_POINT('Ctrl Pts',(3.90000068451114,-1.63115458712464,0.667938911589952));
#11045=CARTESIAN_POINT('Ctrl Pts',(3.90000068976928,-1.6339023205034,0.664721489040691));
#11046=CARTESIAN_POINT('Ctrl Pts',(3.90000069956116,-1.63901923218135,0.658729908073458));
#11047=CARTESIAN_POINT('Ctrl Pts',(3.9000021571807,-1.64338878348726,0.652110283780478));
#11048=CARTESIAN_POINT('Ctrl Pts',(3.90000267296827,-1.64695081636755,0.645027851744832));
#11049=CARTESIAN_POINT('Ctrl Pts',(3.90000272641596,-1.64731992654249,0.644293945625623));
#11050=CARTESIAN_POINT('Ctrl Pts',(3.90000277224081,-1.64768032438231,0.643555049900053));
#11051=CARTESIAN_POINT('Ctrl Pts',(3.90000280957334,-1.64803191324525,0.642811337026806));
#11052=CARTESIAN_POINT('Ctrl Pts',(3.90000316967295,-1.65142324611312,0.635637680016741));
#11053=CARTESIAN_POINT('Ctrl Pts',(3.90000247513984,-1.65395957542788,0.628100801230905));
#11054=CARTESIAN_POINT('Ctrl Pts',(3.90000142932204,-1.65558732484325,0.62036898832433));
#11055=CARTESIAN_POINT('Ctrl Pts',(3.90000076044003,-1.65662839749185,0.615423891207338));
#11056=CARTESIAN_POINT('Ctrl Pts',(3.9,-1.65729694754734,0.61039839235075));
#11057=CARTESIAN_POINT('Ctrl Pts',(3.9,-1.657567947596,0.605334330700044));
#11058=CARTESIAN_POINT('',(3.9,1.55753217754922,0.7));
#11059=CARTESIAN_POINT('',(3.9,0.883148148148148,0.7));
#11060=CARTESIAN_POINT('',(3.9,1.657567947596,0.605334330700044));
#11061=CARTESIAN_POINT('Ctrl Pts',(3.9,1.657567947596,0.605334330700044));
#11062=CARTESIAN_POINT('Ctrl Pts',(3.9,1.65714453107083,0.613246533660879));
#11063=CARTESIAN_POINT('Ctrl Pts',(3.90000169450566,1.65575314729854,0.621067109624563));
#11064=CARTESIAN_POINT('Ctrl Pts',(3.900002426785,1.653477907766,0.628635640467799));
#11065=CARTESIAN_POINT('Ctrl Pts',(3.90000283370343,1.65221358571927,0.632841378048222));
#11066=CARTESIAN_POINT('Ctrl Pts',(3.90000300372053,1.65067534627202,0.636969322077829));
#11067=CARTESIAN_POINT('Ctrl Pts',(3.90000288278183,1.6488710006323,0.640990000951852));
#11068=CARTESIAN_POINT('Ctrl Pts',(3.90000266510116,1.6456233127241,0.64822692378658));
#11069=CARTESIAN_POINT('Ctrl Pts',(3.90000136145047,1.64155197609259,0.655037842274187));
#11070=CARTESIAN_POINT('Ctrl Pts',(3.9000008487987,1.63672139510901,0.661259788874982));
#11071=CARTESIAN_POINT('Ctrl Pts',(3.90000075195303,1.63580884415802,0.662435184403355));
#11072=CARTESIAN_POINT('Ctrl Pts',(3.90000069125178,1.63486906637168,0.663589490553999));
#11073=CARTESIAN_POINT('Ctrl Pts',(3.90000068992127,1.63390232051248,0.664721489040685));
#11074=CARTESIAN_POINT('Ctrl Pts',(3.90000068733544,1.63202347103487,0.666921503393101));
#11075=CARTESIAN_POINT('Ctrl Pts',(3.9000009071255,1.6300427915863,0.669037305429552));
#11076=CARTESIAN_POINT('Ctrl Pts',(3.90000121037842,1.62796736695056,0.671065303566633));
#11077=CARTESIAN_POINT('Ctrl Pts',(3.90000204102081,1.62228255539437,0.676620208836154));
#11078=CARTESIAN_POINT('Ctrl Pts',(3.90000335328325,1.61595386407616,0.681456575151491));
#11079=CARTESIAN_POINT('Ctrl Pts',(3.90000380482706,1.60914557515952,0.685520902406533));
#11080=CARTESIAN_POINT('Ctrl Pts',(3.90000409284089,1.60480295930069,0.688113302965514));
#11081=CARTESIAN_POINT('Ctrl Pts',(3.90000408819389,1.6002642541482,0.690390927291682));
#11082=CARTESIAN_POINT('Ctrl Pts',(3.90000378365133,1.59556629223371,0.692330537597694));
#11083=CARTESIAN_POINT('Ctrl Pts',(3.90000330864444,1.58823869807682,0.695355823328757));
#11084=CARTESIAN_POINT('Ctrl Pts',(3.90000209726118,1.58060840086481,0.697526456028474));
#11085=CARTESIAN_POINT('Ctrl Pts',(3.90000112250675,1.5728228815436,0.698773197673241));
#11086=CARTESIAN_POINT('Ctrl Pts',(3.90000049100668,1.56777898966077,0.699580906164169));
#11087=CARTESIAN_POINT('Ctrl Pts',(3.89999999374416,1.56266934880282,0.69999999924861));
#11088=CARTESIAN_POINT('Ctrl Pts',(3.89999999700315,1.55753217437,0.7));
#11089=CARTESIAN_POINT('Ctrl Pts',(3.9,1.68995649764597,0.));
#11090=CARTESIAN_POINT('Ctrl Pts',(3.9,1.68454744095908,0.101111134163871));
#11091=CARTESIAN_POINT('Ctrl Pts',(3.9,1.67913787721413,0.202223216861756));
#11092=CARTESIAN_POINT('Ctrl Pts',(3.9,1.66834172806373,0.404000675610066));
#11093=CARTESIAN_POINT('Ctrl Pts',(3.9,1.66295504272671,0.504667995047933));
#11094=CARTESIAN_POINT('Ctrl Pts',(3.9,1.657567947596,0.605334330700044));
#11095=CARTESIAN_POINT('Ctrl Pts',(3.90000000000029,-1.68995649764598,2.25514051876985E-17));
#11096=CARTESIAN_POINT('Ctrl Pts',(3.90375240214247,-1.67935614215062,0.202290156525516));
#11097=CARTESIAN_POINT('Ctrl Pts',(3.90750491350916,-1.66875579641967,0.404580311547879));
#11098=CARTESIAN_POINT('Ctrl Pts',(3.91125753584366,-1.65815546066147,0.606870465045848));
#11099=CARTESIAN_POINT('Ctrl Pts',(2.95719731373254,-1.63434162994996,-0.000186284957671625));
#11100=CARTESIAN_POINT('Ctrl Pts',(2.96263618266967,-1.62374249289717,0.202103577800055));
#11101=CARTESIAN_POINT('Ctrl Pts',(2.96807524459186,-1.6131433886527,0.404393433349269));
#11102=CARTESIAN_POINT('Ctrl Pts',(2.97351444051957,-1.60254429060724,0.606683290324339));
#11103=CARTESIAN_POINT('Ctrl Pts',(2.0151035222252,-1.5373601393942,-0.000515615972119944));
#11104=CARTESIAN_POINT('Ctrl Pts',(2.0222299762717,-1.52676329064944,0.20177372753372));
#11105=CARTESIAN_POINT('Ctrl Pts',(2.02935668076532,-1.51616649670304,0.404063061036967));
#11106=CARTESIAN_POINT('Ctrl Pts',(2.03648357820815,-1.50556972342972,0.606352393906678));
#11107=CARTESIAN_POINT('Ctrl Pts',(1.07355614839761,-1.3885225322474,-0.00102014041634142));
#11108=CARTESIAN_POINT('Ctrl Pts',(1.08237048982668,-1.37792954541675,0.201268457136957));
#11109=CARTESIAN_POINT('Ctrl Pts',(1.09118510562603,-1.36733662501784,0.403557046289628));
#11110=CARTESIAN_POINT('Ctrl Pts',(1.09999999998551,-1.35674377243019,0.605845626932519));
#11111=CARTESIAN_POINT('Ctrl Pts',(1.10000000359112,-1.35674374984279,0.605845627045242));
#11112=CARTESIAN_POINT('Ctrl Pts',(2.02777573897866,-1.50422778688462,0.60559460123127));
#11113=CARTESIAN_POINT('Ctrl Pts',(2.96295221054883,-1.60165319397541,0.605428415101273));
#11114=CARTESIAN_POINT('Ctrl Pts',(3.9,-1.657567947596,0.605334330700044));
#11115=CARTESIAN_POINT('Ctrl Pts',(3.90594750914669,-1.55788759822396,0.7));
#11116=CARTESIAN_POINT('Ctrl Pts',(2.96654482017732,-1.50183737247472,0.7));
#11117=CARTESIAN_POINT('Ctrl Pts',(2.02939151553635,-1.40396309164617,0.7));
#11118=CARTESIAN_POINT('Ctrl Pts',(1.1,-1.25565664448621,0.7));
#11119=CARTESIAN_POINT('Ctrl Pts',(3.90422602671531,-1.58673967158186,0.7));
#11120=CARTESIAN_POINT('Ctrl Pts',(2.9639697519154,-1.53062009474021,0.699999324449154));
#11121=CARTESIAN_POINT('Ctrl Pts',(2.02587169016863,-1.43262076012027,0.700001792708215));
#11122=CARTESIAN_POINT('Ctrl Pts',(1.09546090287069,-1.28410178925883,0.700000000000001));
#11123=CARTESIAN_POINT('Ctrl Pts',(3.90124198563808,-1.6367522482393,0.676652244116846));
#11124=CARTESIAN_POINT('Ctrl Pts',(2.95951584878018,-1.58051528054544,0.676683243227538));
#11125=CARTESIAN_POINT('Ctrl Pts',(2.01975879699698,-1.48229505764113,0.676737195552829));
#11126=CARTESIAN_POINT('Ctrl Pts',(1.08759175402576,-1.33341535796084,0.676819902351873));
#11127=CARTESIAN_POINT('Ctrl Pts',(3.90006887217438,-1.65641364884095,0.626981005337021));
#11128=CARTESIAN_POINT('Ctrl Pts',(2.95775794493813,-1.6001648299169,0.627061170854983));
#11129=CARTESIAN_POINT('Ctrl Pts',(2.01735267249256,-1.50192280897576,0.627202240820629));
#11130=CARTESIAN_POINT('Ctrl Pts',(1.08446813262788,-1.35299014570964,0.627416665943555));
#11131=CARTESIAN_POINT('Ctrl Pts',(3.9,-1.657567947596,0.605334330700044));
#11132=CARTESIAN_POINT('Ctrl Pts',(2.95765589353472,-1.60133715645388,0.605428946878649));
#11133=CARTESIAN_POINT('Ctrl Pts',(2.01720431860088,-1.50312513840151,0.605596482146283));
#11134=CARTESIAN_POINT('Ctrl Pts',(1.0842689834292,-1.35423815332579,0.605849891671036));
#11135=CARTESIAN_POINT('Ctrl Pts',(3.89999999700313,-1.55753217437,0.7));
#11136=CARTESIAN_POINT('Ctrl Pts',(2.96258932077475,-1.50142404037792,0.7));
#11137=CARTESIAN_POINT('Ctrl Pts',(2.02743012901897,-1.40365010593343,0.7));
#11138=CARTESIAN_POINT('Ctrl Pts',(1.1,-1.25565664448621,0.7));
#11139=CARTESIAN_POINT('Origin',(6.08012166120517,1.06778195214465E-16,
0.7));
#11140=CARTESIAN_POINT('Ctrl Pts',(1.1,1.25565664448621,0.7));
#11141=CARTESIAN_POINT('Ctrl Pts',(2.02743012901899,1.40365010593344,0.7));
#11142=CARTESIAN_POINT('Ctrl Pts',(2.96258932077472,1.50142404037792,0.7));
#11143=CARTESIAN_POINT('Ctrl Pts',(3.89999999700315,1.55753217437,0.7));
#11144=CARTESIAN_POINT('Ctrl Pts',(1.1,1.25565664448621,0.7));
#11145=CARTESIAN_POINT('Ctrl Pts',(2.02939151553637,1.40396309164617,0.7));
#11146=CARTESIAN_POINT('Ctrl Pts',(2.96654482017727,1.50183737247472,0.7));
#11147=CARTESIAN_POINT('Ctrl Pts',(3.90594750914669,1.55788759822396,0.7));
#11148=CARTESIAN_POINT('Ctrl Pts',(1.09546090287069,1.28410178925883,0.700000000000001));
#11149=CARTESIAN_POINT('Ctrl Pts',(2.02587169016866,1.43262076012027,0.700001792708215));
#11150=CARTESIAN_POINT('Ctrl Pts',(2.96396975191535,1.53062009474021,0.699999324449154));
#11151=CARTESIAN_POINT('Ctrl Pts',(3.90422602671531,1.58673967158186,0.7));
#11152=CARTESIAN_POINT('Ctrl Pts',(1.08759175402576,1.33341535796084,0.676819902351873));
#11153=CARTESIAN_POINT('Ctrl Pts',(2.019758796997,1.48229505764113,0.676737195552829));
#11154=CARTESIAN_POINT('Ctrl Pts',(2.95951584878014,1.58051528054544,0.676683243227538));
#11155=CARTESIAN_POINT('Ctrl Pts',(3.90124198563808,1.6367522482393,0.676652244116846));
#11156=CARTESIAN_POINT('Ctrl Pts',(1.08446813262788,1.35299014570964,0.627416665943555));
#11157=CARTESIAN_POINT('Ctrl Pts',(2.01735267249258,1.50192280897576,0.627202240820629));
#11158=CARTESIAN_POINT('Ctrl Pts',(2.95775794493809,1.6001648299169,0.627061170854983));
#11159=CARTESIAN_POINT('Ctrl Pts',(3.90006887217438,1.65641364884095,0.626981005337021));
#11160=CARTESIAN_POINT('Ctrl Pts',(1.0842689834292,1.35423815332579,0.605849891671036));
#11161=CARTESIAN_POINT('Ctrl Pts',(2.0172043186009,1.50312513840152,0.605596482146283));
#11162=CARTESIAN_POINT('Ctrl Pts',(2.95765589353468,1.60133715645387,0.605428946878649));
#11163=CARTESIAN_POINT('Ctrl Pts',(3.9,1.657567947596,0.605334330700044));
#11164=CARTESIAN_POINT('Ctrl Pts',(3.9,1.657567947596,0.605334330700044));
#11165=CARTESIAN_POINT('Ctrl Pts',(2.96295221054879,1.60165319397541,0.605428415101273));
#11166=CARTESIAN_POINT('Ctrl Pts',(2.02777573897867,1.50422778688462,0.60559460123127));
#11167=CARTESIAN_POINT('Ctrl Pts',(1.10000000359111,1.35674374984279,0.605845627045242));
#11168=CARTESIAN_POINT('Ctrl Pts',(1.07355614839761,1.3885225322474,-0.00102014041634139));
#11169=CARTESIAN_POINT('Ctrl Pts',(1.08237048982668,1.37792954541676,0.201268457136957));
#11170=CARTESIAN_POINT('Ctrl Pts',(1.09118510562602,1.36733662501784,0.403557046289628));
#11171=CARTESIAN_POINT('Ctrl Pts',(1.09999999998551,1.35674377243019,0.605845626932519));
#11172=CARTESIAN_POINT('Ctrl Pts',(2.0151035222252,1.5373601393942,-0.000515615972119942));
#11173=CARTESIAN_POINT('Ctrl Pts',(2.0222299762717,1.52676329064944,0.201773727533721));
#11174=CARTESIAN_POINT('Ctrl Pts',(2.02935668076532,1.51616649670304,0.404063061036968));
#11175=CARTESIAN_POINT('Ctrl Pts',(2.03648357820815,1.50556972342972,0.606352393906678));
#11176=CARTESIAN_POINT('Ctrl Pts',(2.95719731373254,1.63434162994996,-0.000186284957671606));
#11177=CARTESIAN_POINT('Ctrl Pts',(2.96263618266967,1.62374249289717,0.202103577800055));
#11178=CARTESIAN_POINT('Ctrl Pts',(2.96807524459186,1.6131433886527,0.404393433349269));
#11179=CARTESIAN_POINT('Ctrl Pts',(2.97351444051957,1.60254429060724,0.60668329032434));
#11180=CARTESIAN_POINT('Ctrl Pts',(3.90000000000029,1.68995649764598,4.33680868994202E-17));
#11181=CARTESIAN_POINT('Ctrl Pts',(3.90375240214247,1.67935614215062,0.202290156525516));
#11182=CARTESIAN_POINT('Ctrl Pts',(3.90750491350917,1.66875579641967,0.404580311547879));
#11183=CARTESIAN_POINT('Ctrl Pts',(3.91125753584366,1.65815546066147,0.606870465045848));
#11184=CARTESIAN_POINT('Origin',(0.9,1.44962962962963,0.));
#11185=CARTESIAN_POINT('',(0.900000000000025,-1.32415632515176,0.605901073595307));
#11186=CARTESIAN_POINT('Ctrl Pts',(0.900000000000025,-1.32415632515176,
0.605901073595307));
#11187=CARTESIAN_POINT('Ctrl Pts',(0.900000000000025,-1.33021622058432,
0.504787384877132));
#11188=CARTESIAN_POINT('Ctrl Pts',(0.900000000000001,-1.33627289299046,
0.403672458220672));
#11189=CARTESIAN_POINT('Ctrl Pts',(0.900000000000001,-1.3483639425303,0.201706128802639));
#11190=CARTESIAN_POINT('Ctrl Pts',(0.9,-1.3543984610184,0.100852646477479));
#11191=CARTESIAN_POINT('Ctrl Pts',(0.9,-1.3604297237941,0.));
#11192=CARTESIAN_POINT('',(0.9,-1.22294421121193,0.7));
#11193=CARTESIAN_POINT('Ctrl Pts',(0.899999998934589,-1.2229442093848,0.7));
#11194=CARTESIAN_POINT('Ctrl Pts',(0.89999998269596,-1.2309559991361,0.699999991698178));
#11195=CARTESIAN_POINT('Ctrl Pts',(0.900003161357076,-1.2389110096839,0.699008412490225));
#11196=CARTESIAN_POINT('Ctrl Pts',(0.900005837532895,-1.24666554379878,
0.697120920272419));
#11197=CARTESIAN_POINT('Ctrl Pts',(0.900007138246235,-1.25043451364619,
0.69620353424371));
#11198=CARTESIAN_POINT('Ctrl Pts',(0.900008321383585,-1.25415610217771,
0.695073675615989));
#11199=CARTESIAN_POINT('Ctrl Pts',(0.900009136546862,-1.25781268161099,
0.69373809091454));
#11200=CARTESIAN_POINT('Ctrl Pts',(0.90001081442992,-1.26533916477404,0.690989003700189));
#11201=CARTESIAN_POINT('Ctrl Pts',(0.900010659344479,-1.27251458345821,
0.687399440976464));
#11202=CARTESIAN_POINT('Ctrl Pts',(0.900008585023094,-1.27919110928202,
0.68304500924512));
#11203=CARTESIAN_POINT('Ctrl Pts',(0.900007251085311,-1.28348459539356,
0.680244796581297));
#11204=CARTESIAN_POINT('Ctrl Pts',(0.900005156998288,-1.28757155292352,
0.67712723751572));
#11205=CARTESIAN_POINT('Ctrl Pts',(0.900003422242992,-1.29140570811059,
0.673703384872626));
#11206=CARTESIAN_POINT('Ctrl Pts',(0.90000203719427,-1.29446694202502,0.670969741262059));
#11207=CARTESIAN_POINT('Ctrl Pts',(0.90000088611098,-1.29734878548314,0.668056850549005));
#11208=CARTESIAN_POINT('Ctrl Pts',(0.900000936626746,-1.30003070819003,
0.664973821719563));
#11209=CARTESIAN_POINT('Ctrl Pts',(0.90000103432908,-1.30521780373233,0.659010948495488));
#11210=CARTESIAN_POINT('Ctrl Pts',(0.900005119671874,-1.30966005175478,
0.652412896960716));
#11211=CARTESIAN_POINT('Ctrl Pts',(0.900006662646281,-1.31329014967729,
0.64534035177384));
#11212=CARTESIAN_POINT('Ctrl Pts',(0.900006837929091,-1.31370253096037,
0.644536906434065));
#11213=CARTESIAN_POINT('Ctrl Pts',(0.900006988901759,-1.3141043809937,0.64372731654354));
#11214=CARTESIAN_POINT('Ctrl Pts',(0.900007112770807,-1.31449556093743,
0.642911804846506));
#11215=CARTESIAN_POINT('Ctrl Pts',(0.900008198175579,-1.31792328224658,
0.635765868899185));
#11216=CARTESIAN_POINT('Ctrl Pts',(0.900006415208278,-1.32049402672979,
0.628253543462219));
#11217=CARTESIAN_POINT('Ctrl Pts',(0.900003664797616,-1.32215034643222,
0.620540220943237));
#11218=CARTESIAN_POINT('Ctrl Pts',(0.900001948338234,-1.32318401225236,
0.615726538031782));
#11219=CARTESIAN_POINT('Ctrl Pts',(0.900000000000001,-1.32386068836271,
0.610833984830158));
#11220=CARTESIAN_POINT('Ctrl Pts',(0.900000000000001,-1.32415632515176,
0.605901073595307));
#11221=CARTESIAN_POINT('',(0.9,1.22294421121193,0.7));
#11222=CARTESIAN_POINT('',(0.9,0.724814814814815,0.7));
#11223=CARTESIAN_POINT('',(0.900000000000027,1.32415632515176,0.605901073595307));
#11224=CARTESIAN_POINT('Ctrl Pts',(0.900000000000001,1.32415632515176,0.605901073595307));
#11225=CARTESIAN_POINT('Ctrl Pts',(0.900000000000001,1.32368299187747,0.613798977756921));
#11226=CARTESIAN_POINT('Ctrl Pts',(0.900004523569871,1.32223544152535,0.621596324701597));
#11227=CARTESIAN_POINT('Ctrl Pts',(0.900006356724635,1.31990036466821,0.629134362570908));
#11228=CARTESIAN_POINT('Ctrl Pts',(0.900007328861843,1.3186620540024,0.633131846706937));
#11229=CARTESIAN_POINT('Ctrl Pts',(0.900007702029268,1.31717322147439,0.637056437951431));
#11230=CARTESIAN_POINT('Ctrl Pts',(0.900007358328755,1.31544117393516,0.640882963165587));
#11231=CARTESIAN_POINT('Ctrl Pts',(0.900006707239278,1.31216006761937,0.648131745755711));
#11232=CARTESIAN_POINT('Ctrl Pts',(0.900003091243194,1.3080468004769,0.654946293188228));
#11233=CARTESIAN_POINT('Ctrl Pts',(0.900001489347898,1.30317324258861,0.661167512355852));
#11234=CARTESIAN_POINT('Ctrl Pts',(0.900001155878064,1.30215870403359,0.662462596327245));
#11235=CARTESIAN_POINT('Ctrl Pts',(0.90000093695446,1.30111105636563,0.663731893727214));
#11236=CARTESIAN_POINT('Ctrl Pts',(0.90000091848414,1.30003070515708,0.664973821721807));
#11237=CARTESIAN_POINT('Ctrl Pts',(0.90000089007412,1.29836896897911,0.666884086330845));
#11238=CARTESIAN_POINT('Ctrl Pts',(0.900001333486324,1.29662987445651,0.668729618924651));
#11239=CARTESIAN_POINT('Ctrl Pts',(0.900001997973453,1.2948182721625,0.670508241825176));
#11240=CARTESIAN_POINT('Ctrl Pts',(0.900004083621534,1.28913213515815,0.676090865298813));
#11241=CARTESIAN_POINT('Ctrl Pts',(0.900007925915178,1.28279871831387,0.680954424681199));
#11242=CARTESIAN_POINT('Ctrl Pts',(0.900009431597099,1.27598654051802,0.685053039288488));
#11243=CARTESIAN_POINT('Ctrl Pts',(0.900010426918848,1.2714833923965,0.687762403198649));
#11244=CARTESIAN_POINT('Ctrl Pts',(0.900010579450444,1.26676996242859,0.690136867340003));
#11245=CARTESIAN_POINT('Ctrl Pts',(0.900009885932263,1.26188774903006,0.692153145632694));
#11246=CARTESIAN_POINT('Ctrl Pts',(0.900008832351734,1.25447077696631,0.695216239878874));
#11247=CARTESIAN_POINT('Ctrl Pts',(0.900005746465811,1.24674633448708,0.697421320974322));
#11248=CARTESIAN_POINT('Ctrl Pts',(0.900003140090462,1.23886595492982,0.6987028844583));
#11249=CARTESIAN_POINT('Ctrl Pts',(0.900001403206082,1.23361448254879,0.699556916322089));
#11250=CARTESIAN_POINT('Ctrl Pts',(0.899999988093253,1.22829309040712,0.699999994457486));
#11251=CARTESIAN_POINT('Ctrl Pts',(0.899999998934588,1.2229442093848,0.7));
#11252=CARTESIAN_POINT('Ctrl Pts',(0.9,1.3604297237941,0.));
#11253=CARTESIAN_POINT('Ctrl Pts',(0.9,1.35439838926384,0.100853846331769));
#11254=CARTESIAN_POINT('Ctrl Pts',(0.9,1.34836379894337,0.201708528537181));
#11255=CARTESIAN_POINT('Ctrl Pts',(0.9,1.33627274925098,0.403674857922336));
#11256=CARTESIAN_POINT('Ctrl Pts',(0.900000000000027,1.33021614867672,0.504788584706939));
#11257=CARTESIAN_POINT('Ctrl Pts',(0.900000000000027,1.32415632515176,0.605901073595307));
#11258=CARTESIAN_POINT('Ctrl Pts',(0.900000000000001,-1.3604297237941,-1.73472347597681E-18));
#11259=CARTESIAN_POINT('Ctrl Pts',(0.909119345746934,-1.34984469470005,
0.202150401646216));
#11260=CARTESIAN_POINT('Ctrl Pts',(0.918238975454288,-1.33925973741039,
0.404300794324169));
#11261=CARTESIAN_POINT('Ctrl Pts',(0.92735889343571,-1.32867485341111,0.606451177918334));
#11262=CARTESIAN_POINT('Ctrl Pts',(0.693791632045388,-1.32642527651154,
-0.000115194085079675));
#11263=CARTESIAN_POINT('Ctrl Pts',(0.703280422539661,-1.31584113310577,
0.202035038813999));
#11264=CARTESIAN_POINT('Ctrl Pts',(0.712769508818954,-1.30525706820637,
0.404185262036053));
#11265=CARTESIAN_POINT('Ctrl Pts',(0.722258895242942,-1.29467308328318,
0.606335475483814));
#11266=CARTESIAN_POINT('Ctrl Pts',(0.487608314405001,-1.28990207050556,
-0.000238777108575344));
#11267=CARTESIAN_POINT('Ctrl Pts',(0.497466558273561,-1.27931888757273,
0.201911276725417));
#11268=CARTESIAN_POINT('Ctrl Pts',(0.507325109482935,-1.26873579028159,
0.404061320158324));
#11269=CARTESIAN_POINT('Ctrl Pts',(0.517183972542757,-1.25815278023897,
0.606211353085106));
#11270=CARTESIAN_POINT('Ctrl Pts',(0.281447431601629,-1.2507496025167,-0.000370926150909055));
#11271=CARTESIAN_POINT('Ctrl Pts',(0.291675125201343,-1.24016745708839,
0.201778938960696));
#11272=CARTESIAN_POINT('Ctrl Pts',(0.301903137322998,-1.2295854048496,0.403928792940867));
#11273=CARTESIAN_POINT('Ctrl Pts',(0.312131472716966,-1.21900344770756,
0.606078635650713));
#11274=CARTESIAN_POINT('',(0.313137632044026,-1.21919552599285,0.606079286803921));
#11275=CARTESIAN_POINT('Ctrl Pts',(0.28146619846596,-1.25073018526678,-6.36968776335234E-17));
#11276=CARTESIAN_POINT('Ctrl Pts',(0.292023490345879,-1.2402182973453,0.20202640462578));
#11277=CARTESIAN_POINT('Ctrl Pts',(0.302580635585432,-1.22970674279184,
0.404052833452346));
#11278=CARTESIAN_POINT('Ctrl Pts',(0.313137632044028,-1.21919552599286,
0.606079286803922));
#11279=CARTESIAN_POINT('Ctrl Pts',(0.313137632044026,-1.21919552599285,
0.606079286803921));
#11280=CARTESIAN_POINT('Ctrl Pts',(0.508347756773358,-1.25646926692181,
0.606016122348466));
#11281=CARTESIAN_POINT('Ctrl Pts',(0.703992099548353,-1.29143758865737,
0.605956720831638));
#11282=CARTESIAN_POINT('Ctrl Pts',(0.900000000000031,-1.32415632515176,
0.605901073595307));
#11283=CARTESIAN_POINT('Ctrl Pts',(0.916434425702686,-1.22569269236154,
0.7));
#11284=CARTESIAN_POINT('Ctrl Pts',(0.72117838049967,-1.193102781986,0.7));
#11285=CARTESIAN_POINT('Ctrl Pts',(0.526295996270969,-1.15827411715321,
0.7));
#11286=CARTESIAN_POINT('Ctrl Pts',(0.3318563713692,-1.12115139781564,0.7));
#11287=CARTESIAN_POINT('Ctrl Pts',(0.911693828447622,-1.25409504944868,
0.700000000000001));
#11288=CARTESIAN_POINT('Ctrl Pts',(0.716221724293519,-1.22145811194286,
0.699999606692487));
#11289=CARTESIAN_POINT('Ctrl Pts',(0.52112301919326,-1.18657973614434,0.700000445015345));
#11290=CARTESIAN_POINT('Ctrl Pts',(0.32646265058614,-1.14940237362229,0.699999999999999));
#11291=CARTESIAN_POINT('Ctrl Pts',(0.903473253113197,-1.30334701150065,
0.676847307332805));
#11292=CARTESIAN_POINT('Ctrl Pts',(0.707628846166824,-1.27063023858114,
0.676865462359186));
#11293=CARTESIAN_POINT('Ctrl Pts',(0.512149925983835,-1.23566412474798,
0.676884474751893));
#11294=CARTESIAN_POINT('Ctrl Pts',(0.317109102097966,-1.19839394783867,
0.676905055067496));
#11295=CARTESIAN_POINT('Ctrl Pts',(0.900209809599689,-1.32289929215588,
0.627459885485154));
#11296=CARTESIAN_POINT('Ctrl Pts',(0.704212910592823,-1.29017057588713,
0.627506965865002));
#11297=CARTESIAN_POINT('Ctrl Pts',(0.50858160780484,-1.25519230329596,0.627556915196293));
#11298=CARTESIAN_POINT('Ctrl Pts',(0.31338355686088,-1.21790743260971,0.627610331402299));
#11299=CARTESIAN_POINT('Ctrl Pts',(0.900000000000031,-1.32415632515176,
0.605901073595307));
#11300=CARTESIAN_POINT('Ctrl Pts',(0.703992099548353,-1.29143758865737,
0.605956720831638));
#11301=CARTESIAN_POINT('Ctrl Pts',(0.508347756773358,-1.25646926692181,
0.606016122348466));
#11302=CARTESIAN_POINT('Ctrl Pts',(0.313137632044026,-1.21919552599285,
0.606079286803921));
#11303=CARTESIAN_POINT('',(0.3318563713692,-1.12115139781563,0.7));
#11304=CARTESIAN_POINT('Origin',(0.331856371369202,-1.12115139781563,0.6));
#11305=CARTESIAN_POINT('Ctrl Pts',(0.899999998934586,-1.2229442093848,0.7));
#11306=CARTESIAN_POINT('Ctrl Pts',(0.71024282334811,-1.19114655107378,0.7));
#11307=CARTESIAN_POINT('Ctrl Pts',(0.520840466228891,-1.15723253876768,
0.7));
#11308=CARTESIAN_POINT('Ctrl Pts',(0.3318563713692,-1.12115139781564,0.7));
#11309=CARTESIAN_POINT('Origin',(6.08012166120517,1.06778195214465E-16,
0.7));
#11310=CARTESIAN_POINT('',(0.331856371369203,1.12115139781563,0.7));
#11311=CARTESIAN_POINT('',(0.3318563713692,-0.7,0.7));
#11312=CARTESIAN_POINT('Ctrl Pts',(0.331856371369202,1.12115139781564,0.7));
#11313=CARTESIAN_POINT('Ctrl Pts',(0.520840466228894,1.15723253876768,0.7));
#11314=CARTESIAN_POINT('Ctrl Pts',(0.710242823348114,1.19114655107378,0.7));
#11315=CARTESIAN_POINT('Ctrl Pts',(0.899999998934589,1.2229442093848,0.7));
#11316=CARTESIAN_POINT('Ctrl Pts',(0.281447431601628,1.2507496025167,-0.000370926150909064));
#11317=CARTESIAN_POINT('Ctrl Pts',(0.291675125201342,1.24016745708839,0.201778938960695));
#11318=CARTESIAN_POINT('Ctrl Pts',(0.301903137322998,1.2295854048496,0.403928792940867));
#11319=CARTESIAN_POINT('Ctrl Pts',(0.312131472716965,1.21900344770756,0.606078635650713));
#11320=CARTESIAN_POINT('Ctrl Pts',(0.487608314405001,1.28990207050556,-0.000238777108575355));
#11321=CARTESIAN_POINT('Ctrl Pts',(0.497466558273561,1.27931888757273,0.201911276725417));
#11322=CARTESIAN_POINT('Ctrl Pts',(0.507325109482935,1.26873579028159,0.404061320158324));
#11323=CARTESIAN_POINT('Ctrl Pts',(0.517183972542757,1.25815278023897,0.606211353085106));
#11324=CARTESIAN_POINT('Ctrl Pts',(0.693791632045388,1.32642527651154,-0.000115194085079627));
#11325=CARTESIAN_POINT('Ctrl Pts',(0.703280422539661,1.31584113310577,0.202035038813999));
#11326=CARTESIAN_POINT('Ctrl Pts',(0.712769508818955,1.30525706820637,0.404185262036054));
#11327=CARTESIAN_POINT('Ctrl Pts',(0.722258895242942,1.29467308328318,0.606335475483814));
#11328=CARTESIAN_POINT('Ctrl Pts',(0.900000000000002,1.3604297237941,4.33680868994202E-17));
#11329=CARTESIAN_POINT('Ctrl Pts',(0.909119345746935,1.34984469470005,0.202150401646216));
#11330=CARTESIAN_POINT('Ctrl Pts',(0.918238975454289,1.33925973741039,0.40430079432417));
#11331=CARTESIAN_POINT('Ctrl Pts',(0.927358893435711,1.32867485341111,0.606451177918334));
#11332=CARTESIAN_POINT('',(0.313137632044028,1.21919552599286,0.606079286803921));
#11333=CARTESIAN_POINT('Ctrl Pts',(0.900000000000026,1.32415632515176,0.605901073595307));
#11334=CARTESIAN_POINT('Ctrl Pts',(0.703992099548352,1.29143758865737,0.605956720831638));
#11335=CARTESIAN_POINT('Ctrl Pts',(0.508347756773358,1.25646926692181,0.606016122348466));
#11336=CARTESIAN_POINT('Ctrl Pts',(0.313137632044028,1.21919552599286,0.606079286803921));
#11337=CARTESIAN_POINT('Ctrl Pts',(0.313137632044028,1.21919552599286,0.606079286803922));
#11338=CARTESIAN_POINT('Ctrl Pts',(0.302580635585432,1.22970674279184,0.404052833452346));
#11339=CARTESIAN_POINT('Ctrl Pts',(0.29202349034588,1.2402182973453,0.20202640462578));
#11340=CARTESIAN_POINT('Ctrl Pts',(0.28146619846596,1.25073018526678,-6.5594231435373E-18));
#11341=CARTESIAN_POINT('Ctrl Pts',(0.331856371369202,1.12115139781564,0.7));
#11342=CARTESIAN_POINT('Ctrl Pts',(0.526295996270969,1.15827411715321,0.7));
#11343=CARTESIAN_POINT('Ctrl Pts',(0.72117838049967,1.193102781986,0.7));
#11344=CARTESIAN_POINT('Ctrl Pts',(0.916434425702682,1.22569269236154,0.7));
#11345=CARTESIAN_POINT('Ctrl Pts',(0.326462650586141,1.14940237362229,0.699999999999999));
#11346=CARTESIAN_POINT('Ctrl Pts',(0.52112301919326,1.18657973614434,0.700000445015345));
#11347=CARTESIAN_POINT('Ctrl Pts',(0.716221724293519,1.22145811194286,0.699999606692487));
#11348=CARTESIAN_POINT('Ctrl Pts',(0.911693828447618,1.25409504944868,0.700000000000001));
#11349=CARTESIAN_POINT('Ctrl Pts',(0.317109102097967,1.19839394783867,0.676905055067496));
#11350=CARTESIAN_POINT('Ctrl Pts',(0.512149925983836,1.23566412474798,0.676884474751893));
#11351=CARTESIAN_POINT('Ctrl Pts',(0.707628846166824,1.27063023858114,0.676865462359185));
#11352=CARTESIAN_POINT('Ctrl Pts',(0.903473253113193,1.30334701150065,0.676847307332805));
#11353=CARTESIAN_POINT('Ctrl Pts',(0.313383556860882,1.21790743260971,0.627610331402299));
#11354=CARTESIAN_POINT('Ctrl Pts',(0.508581607804839,1.25519230329596,0.627556915196293));
#11355=CARTESIAN_POINT('Ctrl Pts',(0.704212910592822,1.29017057588713,0.627506965865002));
#11356=CARTESIAN_POINT('Ctrl Pts',(0.900209809599685,1.32289929215587,0.627459885485154));
#11357=CARTESIAN_POINT('Ctrl Pts',(0.313137632044028,1.21919552599286,0.606079286803921));
#11358=CARTESIAN_POINT('Ctrl Pts',(0.508347756773358,1.25646926692181,0.606016122348466));
#11359=CARTESIAN_POINT('Ctrl Pts',(0.703992099548352,1.29143758865737,0.605956720831638));
#11360=CARTESIAN_POINT('Ctrl Pts',(0.900000000000026,1.32415632515176,0.605901073595307));
#11361=CARTESIAN_POINT('Origin',(0.3318563713692,1.12115139781563,0.6));
#11362=CARTESIAN_POINT('Origin',(0.3318563713692,1.12115139781563,0.6));
#11363=CARTESIAN_POINT('Origin',(0.3318563713692,1.12115139781563,0.6));
#11364=CARTESIAN_POINT('Origin',(0.331856371369201,1.12115139781563,0.6));
#11365=CARTESIAN_POINT('Origin',(11.6681436286308,1.2964346619681,0.6));
#11366=CARTESIAN_POINT('Origin',(11.6681436286308,1.2964346619681,0.6));
#11367=CARTESIAN_POINT('',(11.7680065821063,1.2964346619681,0.605233595624295));
#11368=CARTESIAN_POINT('Origin',(11.6681436286308,1.2964346619681,0.6));
#11369=CARTESIAN_POINT('Origin',(11.6681436286308,1.2964346619681,0.6));
#11370=CARTESIAN_POINT('Origin',(0.3318563713692,-1.12115139781563,0.6));
#11371=CARTESIAN_POINT('Origin',(0.3318563713692,-1.12115139781563,0.6));
#11372=CARTESIAN_POINT('Origin',(0.3318563713692,-1.12115139781563,0.6));
#11373=CARTESIAN_POINT('Origin',(0.3318563713692,-0.7,0.6));
#11374=CARTESIAN_POINT('Ctrl Pts',(0.281398851089427,-1.25079724300364,
-0.00128877254616805));
#11375=CARTESIAN_POINT('Ctrl Pts',(0.291978592719145,-1.24026300108396,
0.201167222825305));
#11376=CARTESIAN_POINT('Ctrl Pts',(0.302558187088771,-1.2297290939422,0.403623242499903));
#11377=CARTESIAN_POINT('Ctrl Pts',(0.313137632044028,-1.21919552599286,
0.606079286803922));
#11378=CARTESIAN_POINT('Ctrl Pts',(0.258825925396095,-1.24645021448495,
-0.000331836826913007));
#11379=CARTESIAN_POINT('Ctrl Pts',(0.269412087408768,-1.23590982471973,
0.202123507634926));
#11380=CARTESIAN_POINT('Ctrl Pts',(0.279998097240749,-1.22537010804418,
0.404578894752494));
#11381=CARTESIAN_POINT('Ctrl Pts',(0.290584031570127,-1.21483034200885,
0.60703428203898));
#11382=CARTESIAN_POINT('Ctrl Pts',(0.216858515231733,-1.22156435206688,
0.000573427186746937));
#11383=CARTESIAN_POINT('Ctrl Pts',(0.22746089442761,-1.21102065820065,0.20302778119957));
#11384=CARTESIAN_POINT('Ctrl Pts',(0.238063405890532,-1.20047706879609,
0.405482132943502));
#11385=CARTESIAN_POINT('Ctrl Pts',(0.248665715176951,-1.18993398276804,
0.607936521147589));
#11386=CARTESIAN_POINT('Ctrl Pts',(0.20022524016831,-1.1757120364715,-0.000939345874739115));
#11387=CARTESIAN_POINT('Ctrl Pts',(0.210835545796271,-1.16517845930889,
0.201515175954065));
#11388=CARTESIAN_POINT('Ctrl Pts',(0.221445511453644,-1.15464532122135,
0.403969738345816));
#11389=CARTESIAN_POINT('Ctrl Pts',(0.232055819885544,-1.1441124535127,0.606424296559432));
#11390=CARTESIAN_POINT('Ctrl Pts',(0.200162791320387,-1.15273540576203,
-0.00213094087794781));
#11391=CARTESIAN_POINT('Ctrl Pts',(0.210772999146098,-1.14220702337553,
0.200323884929633));
#11392=CARTESIAN_POINT('Ctrl Pts',(0.221383207999129,-1.13167901896849,
0.402778730339676));
#11393=CARTESIAN_POINT('Ctrl Pts',(0.231993417893744,-1.12115139781563,
0.605233595624295));
#11394=CARTESIAN_POINT('Origin',(11.6681436286308,-1.2964346619681,0.6));
#11395=CARTESIAN_POINT('',(11.7680065821063,-1.2964346619681,0.605233595624295));
#11396=CARTESIAN_POINT('Origin',(11.6681436286308,-1.2964346619681,0.6));
#11397=CARTESIAN_POINT('Origin',(11.6681436286308,-1.2964346619681,0.6));
#11398=CARTESIAN_POINT('Origin',(11.6681436286308,0.8,0.6));
#11399=CARTESIAN_POINT('',(11.7680065821063,0.8,0.605233595624295));
#11400=CARTESIAN_POINT('Ctrl Pts',(11.7998406965532,-1.32812796269332,-0.00219749346969486));
#11401=CARTESIAN_POINT('Ctrl Pts',(11.7892293257052,-1.31756329650235,0.200279524124498));
#11402=CARTESIAN_POINT('Ctrl Pts',(11.778617954226,-1.30699886176745,0.402756553762325));
#11403=CARTESIAN_POINT('Ctrl Pts',(11.7680065821063,-1.2964346619681,0.605233595624295));
#11404=CARTESIAN_POINT('Ctrl Pts',(11.7997644051931,-1.35610429277321,-0.000741767599518841));
#11405=CARTESIAN_POINT('Ctrl Pts',(11.7891529352516,-1.34553639595159,0.201735054786578));
#11406=CARTESIAN_POINT('Ctrl Pts',(11.7785417923834,-1.33496887357233,0.404211913913734));
#11407=CARTESIAN_POINT('Ctrl Pts',(11.7679303202531,-1.32440140973518,0.606688758469115));
#11408=CARTESIAN_POINT('Ctrl Pts',(11.777798894316,-1.40464673224301,0.000639873095493681));
#11409=CARTESIAN_POINT('Ctrl Pts',(11.7671928076068,-1.39407357725403,0.203116666245104));
#11410=CARTESIAN_POINT('Ctrl Pts',(11.7565866683578,-1.38350056680667,0.405593463707878));
#11411=CARTESIAN_POINT('Ctrl Pts',(11.7459806329718,-1.37292778989405,0.608070278434593));
#11412=CARTESIAN_POINT('Ctrl Pts',(11.7305637688674,-1.42539741767755,-0.000752904078362463));
#11413=CARTESIAN_POINT('Ctrl Pts',(11.7199663219939,-1.4148278080644,0.201724510929383));
#11414=CARTESIAN_POINT('Ctrl Pts',(11.7093688723049,-1.40425849106451,0.404201940657439));
#11415=CARTESIAN_POINT('Ctrl Pts',(11.6987715660822,-1.39368929079062,0.606679383299034));
#11416=CARTESIAN_POINT('Ctrl Pts',(11.7096810564041,-1.4274931182575,-0.0017379730583696));
#11417=CARTESIAN_POINT('Ctrl Pts',(11.6990862989954,-1.41692678914967,0.200739752511227));
#11418=CARTESIAN_POINT('Ctrl Pts',(11.6884916259906,-1.40636067879325,0.403217493356832));
#11419=CARTESIAN_POINT('Ctrl Pts',(11.6778970386953,-1.39579479040469,0.605695249702977));
#11420=CARTESIAN_POINT('Ctrl Pts',(11.7997255308004,-1.32801330383774,1.58293517182884E-17));
#11421=CARTESIAN_POINT('Ctrl Pts',(11.7891525485321,-1.31748685893698,0.201744519857947));
#11422=CARTESIAN_POINT('Ctrl Pts',(11.7785795656372,-1.30696064383315,0.403489051673192));
#11423=CARTESIAN_POINT('Ctrl Pts',(11.7680065821063,-1.2964346619681,0.605233595624295));
#11424=CARTESIAN_POINT('Ctrl Pts',(11.7096782931395,1.42749036240749,-0.00168516396645821));
#11425=CARTESIAN_POINT('Ctrl Pts',(11.6990844568337,1.41692495195436,0.200774958575157));
#11426=CARTESIAN_POINT('Ctrl Pts',(11.6884907049172,1.40635976021489,0.403235096390144));
#11427=CARTESIAN_POINT('Ctrl Pts',(11.6778970386953,1.39579479040469,0.605695249702978));
#11428=CARTESIAN_POINT('Ctrl Pts',(11.7375219088137,1.42469609383707,-0.000371738767665111));
#11429=CARTESIAN_POINT('Ctrl Pts',(11.7269244310859,1.41412622652679,0.202087962343291));
#11430=CARTESIAN_POINT('Ctrl Pts',(11.7163270893473,1.40355692684423,0.404547700208143));
#11431=CARTESIAN_POINT('Ctrl Pts',(11.7057297418778,1.39298745758592,0.607007427831054));
#11432=CARTESIAN_POINT('Ctrl Pts',(11.7837126264455,1.39812338730171,0.000662527065309348));
#11433=CARTESIAN_POINT('Ctrl Pts',(11.7731059659782,1.38755170250994,0.203121672627585));
#11434=CARTESIAN_POINT('Ctrl Pts',(11.762499302106,1.37698011891703,0.405580822779681));
#11435=CARTESIAN_POINT('Ctrl Pts',(11.7518926781287,1.36640881816393,0.608039989525598));
#11436=CARTESIAN_POINT('Ctrl Pts',(11.7997807104374,1.34910745421534,-0.00105289019631603));
#11437=CARTESIAN_POINT('Ctrl Pts',(11.7891702365097,1.33854134055748,0.201406383632416));
#11438=CARTESIAN_POINT('Ctrl Pts',(11.7785598611315,1.32797539467558,0.403865671186622));
#11439=CARTESIAN_POINT('Ctrl Pts',(11.7679493857164,1.31740972279341,0.60632496775791));
#11440=CARTESIAN_POINT('Ctrl Pts',(11.7998379289556,1.32812520727701,-0.00214468456243374));
#11441=CARTESIAN_POINT('Ctrl Pts',(11.78922748064,1.31756145959839,0.200314730064766));
#11442=CARTESIAN_POINT('Ctrl Pts',(11.7786170316934,1.30699794333589,0.402774156733522));
#11443=CARTESIAN_POINT('Ctrl Pts',(11.7680065821063,1.2964346619681,0.605233595624295));
#11444=CARTESIAN_POINT('Ctrl Pts',(11.7680065821063,1.2964346619681,0.605233595624295));
#11445=CARTESIAN_POINT('Ctrl Pts',(11.7785795656372,1.30696064383315,0.403489051673192));
#11446=CARTESIAN_POINT('Ctrl Pts',(11.7891525485321,1.31748685893698,0.201744519857946));
#11447=CARTESIAN_POINT('Ctrl Pts',(11.7997255308004,1.32801330383774,3.10081821330854E-17));
#11448=CARTESIAN_POINT('Ctrl Pts',(11.3905090053564,1.32332268868375,0.7));
#11449=CARTESIAN_POINT('Ctrl Pts',(11.4830653488871,1.31448403714216,0.7));
#11450=CARTESIAN_POINT('Ctrl Pts',(11.5756099286391,1.3055179747114,0.7));
#11451=CARTESIAN_POINT('Ctrl Pts',(11.6681436286308,1.2964346619681,0.7));
#11452=CARTESIAN_POINT('Ctrl Pts',(11.3932507170007,1.35203326785047,0.7));
#11453=CARTESIAN_POINT('Ctrl Pts',(11.4858332859074,1.34318985044544,0.699999917777441));
#11454=CARTESIAN_POINT('Ctrl Pts',(11.5784027531871,1.33421922733773,0.700000082825348));
#11455=CARTESIAN_POINT('Ctrl Pts',(11.6709605510772,1.32513126902304,0.7));
#11456=CARTESIAN_POINT('Ctrl Pts',(11.3980029235658,1.40179729139028,0.67675176769038));
#11457=CARTESIAN_POINT('Ctrl Pts',(11.4906306781252,1.39294591144353,0.676755553516685));
#11458=CARTESIAN_POINT('Ctrl Pts',(11.583243842395,1.38396722707511,0.676759299309383));
#11459=CARTESIAN_POINT('Ctrl Pts',(11.6758431636759,1.37487151491717,0.676763114282959));
#11460=CARTESIAN_POINT('Ctrl Pts',(11.3998836071583,1.4214913811319,0.627256563056779));
#11461=CARTESIAN_POINT('Ctrl Pts',(11.4925297866457,1.41264104586547,0.627266369072496));
#11462=CARTESIAN_POINT('Ctrl Pts',(11.5851604051362,1.40366358810601,0.627276165220861));
#11463=CARTESIAN_POINT('Ctrl Pts',(11.6777767156198,1.39456903283364,0.627286048421068));
#11464=CARTESIAN_POINT('Ctrl Pts',(11.4,1.4227102204299,0.605660349289938));
#11465=CARTESIAN_POINT('Ctrl Pts',(11.4926474653491,1.41386220753305,0.605671932550561));
#11466=CARTESIAN_POINT('Ctrl Pts',(11.585279512325,1.40488700096013,0.605683574233495));
#11467=CARTESIAN_POINT('Ctrl Pts',(11.6778970386953,1.39579479040469,0.605695249702977));
#11468=CARTESIAN_POINT('Ctrl Pts',(0.200160078391861,1.15273809776858,-0.00218270663797729));
#11469=CARTESIAN_POINT('Ctrl Pts',(0.210771190526905,1.14220881798213,0.200289374419605));
#11470=CARTESIAN_POINT('Ctrl Pts',(0.221382303689445,1.13167991623912,0.402761475082968));
#11471=CARTESIAN_POINT('Ctrl Pts',(0.231993417893744,1.12115139781563,0.605233595624295));
#11472=CARTESIAN_POINT('Ctrl Pts',(0.200222527243758,1.17571472979894,-0.000991111558954063));
#11473=CARTESIAN_POINT('Ctrl Pts',(0.210833737189325,1.165180254798,0.201480665494204));
#11474=CARTESIAN_POINT('Ctrl Pts',(0.22144460713556,1.15464621893915,0.403952483115279));
#11475=CARTESIAN_POINT('Ctrl Pts',(0.232055819885544,1.1441124535127,0.606424296559433));
#11476=CARTESIAN_POINT('Ctrl Pts',(0.216855804290742,1.22156704800519,0.000521661548984882));
#11477=CARTESIAN_POINT('Ctrl Pts',(0.22745908713481,1.21102245544698,0.202993270772045));
#11478=CARTESIAN_POINT('Ctrl Pts',(0.238062502254218,1.2004779673848,0.405464877727456));
#11479=CARTESIAN_POINT('Ctrl Pts',(0.248665715176951,1.18993398276804,0.607936521147589));
#11480=CARTESIAN_POINT('Ctrl Pts',(0.258823218619159,1.24645290953083,-0.000383602721372307));
#11481=CARTESIAN_POINT('Ctrl Pts',(0.269410282911183,1.23591162135389,0.202088997034388));
#11482=CARTESIAN_POINT('Ctrl Pts',(0.279997195000074,1.22537100634993,0.404561639451295));
#11483=CARTESIAN_POINT('Ctrl Pts',(0.290584031570127,1.21483034200885,0.60703428203898));
#11484=CARTESIAN_POINT('Ctrl Pts',(0.281396145950812,1.25079993650842,-0.00134053860524368));
#11485=CARTESIAN_POINT('Ctrl Pts',(0.291976789318506,1.24026479669674,0.201132712115111));
#11486=CARTESIAN_POINT('Ctrl Pts',(0.302557285401186,1.22972999171968,0.403605987142707));
#11487=CARTESIAN_POINT('Ctrl Pts',(0.313137632044028,1.21919552599286,0.606079286803922));
#11488=CARTESIAN_POINT('Origin',(11.8002740930491,1.6,-0.0104671912485888));
#11489=CARTESIAN_POINT('Origin',(0.3318563713692,1.12115139781563,0.6));
#11490=CARTESIAN_POINT('',(0.331856371369203,1.12115139781563,0.9));
#11491=CARTESIAN_POINT('',(0.0322675109428288,1.12115139781563,0.615700786872883));
#11492=CARTESIAN_POINT('Origin',(0.3318563713692,1.12115139781563,0.6));
#11493=CARTESIAN_POINT('',(0.275700153393682,1.4152837823473,0.618237860411764));
#11494=CARTESIAN_POINT('Origin',(0.3318563713692,1.12115139781563,0.6));
#11495=CARTESIAN_POINT('Origin',(0.331856371369201,1.12115139781563,0.600000000000001));
#11496=CARTESIAN_POINT('Origin',(11.6681436286308,1.2964346619681,0.6));
#11497=CARTESIAN_POINT('',(11.6681436286308,1.2964346619681,0.9));
#11498=CARTESIAN_POINT('',(11.6974038588243,1.59451504727786,0.617085749108931));
#11499=CARTESIAN_POINT('Origin',(11.6681436286308,1.2964346619681,0.6));
#11500=CARTESIAN_POINT('',(11.9677324890572,1.2964346619681,0.615700786872884));
#11501=CARTESIAN_POINT('Origin',(11.6681436286308,1.2964346619681,0.6));
#11502=CARTESIAN_POINT('Origin',(11.6681436286308,1.2964346619681,0.6));
#11503=CARTESIAN_POINT('Origin',(0.3318563713692,-1.12115139781563,0.6));
#11504=CARTESIAN_POINT('',(0.3318563713692,-1.12115139781563,0.9));
#11505=CARTESIAN_POINT('',(0.27570015339368,-1.4152837823473,0.618237860411764));
#11506=CARTESIAN_POINT('Origin',(0.331856371369206,-1.12115139781563,0.6));
#11507=CARTESIAN_POINT('',(0.0322675109428289,-1.12115139781563,0.615700786872884));
#11508=CARTESIAN_POINT('Origin',(0.3318563713692,-1.12115139781563,0.6));
#11509=CARTESIAN_POINT('Origin',(0.331856371369201,-1.12115139781563,0.6));
#11510=CARTESIAN_POINT('Origin',(0.3318563713692,-0.7,0.6));
#11511=CARTESIAN_POINT('',(0.0322675109428288,-0.7,0.615700786872883));
#11512=CARTESIAN_POINT('',(0.3318563713692,-0.7,0.9));
#11513=CARTESIAN_POINT('Ctrl Pts',(0.243379792658812,-1.44768816351885,
-0.00386660544379547));
#11514=CARTESIAN_POINT('Ctrl Pts',(0.254153714020244,-1.43688644166428,
0.203501514337738));
#11515=CARTESIAN_POINT('Ctrl Pts',(0.264927169923045,-1.42608498030896,
0.410869669467268));
#11516=CARTESIAN_POINT('Ctrl Pts',(0.275700153393682,-1.4152837823473,0.618237860411764));
#11517=CARTESIAN_POINT('Ctrl Pts',(0.165985306518657,-1.43278556900406,
-0.000585522405354874));
#11518=CARTESIAN_POINT('Ctrl Pts',(0.176781886982148,-1.42196211044871,
0.206780297826791));
#11519=CARTESIAN_POINT('Ctrl Pts',(0.187577631459021,-1.41114055376332,
0.414146260476818));
#11520=CARTESIAN_POINT('Ctrl Pts',(0.198373523197449,-1.40031743725927,
0.621512129789107));
#11521=CARTESIAN_POINT('Ctrl Pts',(0.0420337764471552,-1.35067831466576,
0.00164062070145552));
#11522=CARTESIAN_POINT('Ctrl Pts',(0.0528811856485653,-1.33984924001505,
0.209003590924217));
#11523=CARTESIAN_POINT('Ctrl Pts',(0.0637288270387668,-1.3290196870647,
0.416366521726085));
#11524=CARTESIAN_POINT('Ctrl Pts',(0.0745760486629849,-1.31819094697801,
0.623729515932473));
#11525=CARTESIAN_POINT('Ctrl Pts',(-0.000174449685670057,-1.21258510413485,
-0.00332869829739982));
#11526=CARTESIAN_POINT('Ctrl Pts',(0.0106931634330696,-1.20178787588112,
0.204035045544629));
#11527=CARTESIAN_POINT('Ctrl Pts',(0.0215603573327632,-1.19099068058357,
0.411398812224037));
#11528=CARTESIAN_POINT('Ctrl Pts',(0.0324279732074593,-1.18019411246525,
0.618762589277523));
#11529=CARTESIAN_POINT('Ctrl Pts',(-0.000335035344191381,-1.15350137313465,
-0.00639285519773308));
#11530=CARTESIAN_POINT('Ctrl Pts',(0.0105324790023165,-1.1427176497384,
0.200971671503832));
#11531=CARTESIAN_POINT('Ctrl Pts',(0.0213999944262164,-1.13193432274319,
0.408336218763261));
#11532=CARTESIAN_POINT('Ctrl Pts',(0.0322675109428286,-1.12115139781563,
0.615700786872884));
#11533=CARTESIAN_POINT('Ctrl Pts',(0.243580684154575,-1.44748675362873,
-2.16840434497101E-17));
#11534=CARTESIAN_POINT('Ctrl Pts',(0.254287635915809,-1.43675217163244,
0.206079251738322));
#11535=CARTESIAN_POINT('Ctrl Pts',(0.264994127943615,-1.42601784692504,
0.412158538389471));
#11536=CARTESIAN_POINT('Ctrl Pts',(0.275700153393682,-1.4152837823473,0.618237860411764));
#11537=CARTESIAN_POINT('Ctrl Pts',(0.0322675109428286,-1.12115139781563,
0.615700786872884));
#11538=CARTESIAN_POINT('Ctrl Pts',(0.0215116728964671,-1.13182351356624,
0.410467170919192));
#11539=CARTESIAN_POINT('Ctrl Pts',(0.0107558359204751,-1.14249602316337,
0.205233575389367));
#11540=CARTESIAN_POINT('Ctrl Pts',(-1.41190227911925E-16,-1.15316892111333,
8.06646416329215E-17));
#11541=CARTESIAN_POINT('Origin',(11.6681436286308,-1.2964346619681,0.6));
#11542=CARTESIAN_POINT('',(11.9677324890572,-1.2964346619681,0.615700786872884));
#11543=CARTESIAN_POINT('',(11.6974038588243,-1.59451504727786,0.617085749108931));
#11544=CARTESIAN_POINT('Origin',(11.6681436286308,-1.2964346619681,0.600000000000001));
#11545=CARTESIAN_POINT('',(11.6681436286308,-1.2964346619681,0.9));
#11546=CARTESIAN_POINT('Origin',(11.6681436286308,-1.2964346619681,0.6));
#11547=CARTESIAN_POINT('Origin',(11.6681436286308,-1.2964346619681,0.6));
#11548=CARTESIAN_POINT('Origin',(11.6681436286308,0.8,0.6));
#11549=CARTESIAN_POINT('',(11.9677324890572,0.8,0.615700786872884));
#11550=CARTESIAN_POINT('',(11.6681436286308,0.8,0.9));
#11551=CARTESIAN_POINT('Ctrl Pts',(11.6681436286308,-1.2964346619681,0.9));
#11552=CARTESIAN_POINT('Ctrl Pts',(10.0505146497799,-1.45522470190849,0.9));
#11553=CARTESIAN_POINT('Ctrl Pts',(7.34698379851713,-1.66064017564263,0.9));
#11554=CARTESIAN_POINT('Ctrl Pts',(3.5507249968367,-1.5921338472202,0.9));
#11555=CARTESIAN_POINT('Ctrl Pts',(1.39628032950236,-1.32437289587156,0.9));
#11556=CARTESIAN_POINT('Ctrl Pts',(0.331856371369199,-1.12115139781563,
0.9));
#11557=CARTESIAN_POINT('Ctrl Pts',(11.6765943959699,-1.38252448313292,0.9));
#11558=CARTESIAN_POINT('Ctrl Pts',(10.0577014803155,-1.54155822929668,0.900004386952174));
#11559=CARTESIAN_POINT('Ctrl Pts',(7.35045927226653,-1.74750661992774,0.90000020513805));
#11560=CARTESIAN_POINT('Ctrl Pts',(3.54497585078588,-1.67885197560093,0.899998846478116));
#11561=CARTESIAN_POINT('Ctrl Pts',(1.38372480803625,-1.41002339692611,0.900007381454799));
#11562=CARTESIAN_POINT('Ctrl Pts',(0.315675209020016,-1.2059043252356,0.9));
#11563=CARTESIAN_POINT('Ctrl Pts',(11.6912432102654,-1.53175516862908,0.830242007927396));
#11564=CARTESIAN_POINT('Ctrl Pts',(10.070172518288,-1.69119563674726,0.830042231904815));
#11565=CARTESIAN_POINT('Ctrl Pts',(7.35645297288469,-1.89806162871739,0.829725685238203));
#11566=CARTESIAN_POINT('Ctrl Pts',(3.53503777381493,-1.8291593714544,0.829829026055289));
#11567=CARTESIAN_POINT('Ctrl Pts',(1.36192166831068,-1.55847530615989,0.830279056498203));
#11568=CARTESIAN_POINT('Ctrl Pts',(0.28762358730286,-1.35283178372728,0.830616544072481));
#11569=CARTESIAN_POINT('Ctrl Pts',(11.6970428895979,-1.59083777456472,0.681858145263203));
#11570=CARTESIAN_POINT('Ctrl Pts',(10.0750816081461,-1.75021732245097,0.681339641080976));
#11571=CARTESIAN_POINT('Ctrl Pts',(7.3588078744758,-1.95708146899443,0.680519979048775));
#11572=CARTESIAN_POINT('Ctrl Pts',(3.53113644431293,-1.88819699008302,0.68078748362792));
#11573=CARTESIAN_POINT('Ctrl Pts',(1.35331700817769,-1.61730376958615,0.681953432622034));
#11574=CARTESIAN_POINT('Ctrl Pts',(0.276437927844241,-1.41141950219787,
0.682830994206899));
#11575=CARTESIAN_POINT('Ctrl Pts',(11.6974038588243,-1.59451504727786,0.617085749108931));
#11576=CARTESIAN_POINT('Ctrl Pts',(10.0753786444688,-1.75377172884558,0.616473434532366));
#11577=CARTESIAN_POINT('Ctrl Pts',(7.35893161235257,-1.96044797105896,0.61550283428964));
#11578=CARTESIAN_POINT('Ctrl Pts',(3.53092277948893,-1.89162724517065,0.615818637525046));
#11579=CARTESIAN_POINT('Ctrl Pts',(1.35277799022997,-1.62098550016515,0.617200513836093));
#11580=CARTESIAN_POINT('Ctrl Pts',(0.27570015339368,-1.4152837823473,0.618237860411764));
#11581=CARTESIAN_POINT('Ctrl Pts',(0.27570015339368,-1.4152837823473,0.618237860411764));
#11582=CARTESIAN_POINT('Ctrl Pts',(1.35277799022997,-1.62098550016515,0.617200513836093));
#11583=CARTESIAN_POINT('Ctrl Pts',(3.53092277948893,-1.89162724517065,0.615818637525046));
#11584=CARTESIAN_POINT('Ctrl Pts',(7.35893161235257,-1.96044797105896,0.61550283428964));
#11585=CARTESIAN_POINT('Ctrl Pts',(10.0753786444688,-1.75377172884558,0.616473434532366));
#11586=CARTESIAN_POINT('Ctrl Pts',(11.6974038588243,-1.59451504727786,0.617085749108931));
#11587=CARTESIAN_POINT('Ctrl Pts',(11.6681436286308,-1.2964346619681,0.9));
#11588=CARTESIAN_POINT('Ctrl Pts',(10.0505146497799,-1.45522470190849,0.9));
#11589=CARTESIAN_POINT('Ctrl Pts',(7.34698379851713,-1.66064017564263,0.9));
#11590=CARTESIAN_POINT('Ctrl Pts',(3.5507249968367,-1.5921338472202,0.9));
#11591=CARTESIAN_POINT('Ctrl Pts',(1.39628032950236,-1.32437289587156,0.9));
#11592=CARTESIAN_POINT('Ctrl Pts',(0.331856371369199,-1.12115139781563,
0.9));
#11593=CARTESIAN_POINT('Ctrl Pts',(12.0003454972153,-1.32890342861544,-0.00659247958978532));
#11594=CARTESIAN_POINT('Ctrl Pts',(11.9894744951615,-1.31808026232082,0.200838596530835));
#11595=CARTESIAN_POINT('Ctrl Pts',(11.9786034924455,-1.30725733885828,0.408269685287046));
#11596=CARTESIAN_POINT('Ctrl Pts',(11.9677324890572,-1.2964346619681,0.615700786872884));
#11597=CARTESIAN_POINT('Ctrl Pts',(12.000116620981,-1.41283311850955,-0.00222526087931226));
#11598=CARTESIAN_POINT('Ctrl Pts',(11.9892453109784,-1.40200002127642,0.205205215027088));
#11599=CARTESIAN_POINT('Ctrl Pts',(11.9783750177566,-1.39116761830557,0.412635780645844));
#11600=CARTESIAN_POINT('Ctrl Pts',(11.9675037034976,-1.38033490526933,0.620066275407343));
#11601=CARTESIAN_POINT('Ctrl Pts',(11.9341774721098,-1.5584705948029,0.00191796595980313));
#11602=CARTESIAN_POINT('Ctrl Pts',(11.9233226835938,-1.54762133657986,0.209348350794306));
#11603=CARTESIAN_POINT('Ctrl Pts',(11.9124678718222,-1.53677206634062,0.416778732304926));
#11604=CARTESIAN_POINT('Ctrl Pts',(11.9016132473252,-1.52592301942363,0.624209134118803));
#11605=CARTESIAN_POINT('Ctrl Pts',(11.7925116537096,-1.62071287545028,-0.0022587989925734));
#11606=CARTESIAN_POINT('Ctrl Pts',(11.7816834491585,-1.6098745265243,0.205173499361722));
#11607=CARTESIAN_POINT('Ctrl Pts',(11.7708551999607,-1.59903658749835,0.41260581547062));
#11608=CARTESIAN_POINT('Ctrl Pts',(11.760027440985,-1.58819854843564,0.620038149897102));
#11609=CARTESIAN_POINT('Ctrl Pts',(11.7298629188572,-1.62699926142283,-0.0052140742384003));
#11610=CARTESIAN_POINT('Ctrl Pts',(11.7190429637906,-1.61617098622686,0.202219177289036));
#11611=CARTESIAN_POINT('Ctrl Pts',(11.708223275703,-1.60534291388117,0.409652451626141));
#11612=CARTESIAN_POINT('Ctrl Pts',(11.6974038588243,-1.59451504727786,0.617085749108931));
#11613=CARTESIAN_POINT('Ctrl Pts',(12.,-1.32855945177638,-1.94722710178397E-16));
#11614=CARTESIAN_POINT('Ctrl Pts',(11.9892441636707,-1.31785094954632,0.205233583190348));
#11615=CARTESIAN_POINT('Ctrl Pts',(11.978488326693,-1.30714268506935,0.410467178751997));
#11616=CARTESIAN_POINT('Ctrl Pts',(11.9677324890572,-1.2964346619681,0.615700786872884));
#11617=CARTESIAN_POINT('Ctrl Pts',(11.6974038588243,-1.59451504727786,0.617085749108931));
#11618=CARTESIAN_POINT('Ctrl Pts',(11.7081326228587,-1.605252190239,0.41139047675572));
#11619=CARTESIAN_POINT('Ctrl Pts',(11.7188616535763,-1.61598953550924,0.205695227161956));
#11620=CARTESIAN_POINT('Ctrl Pts',(11.7295909468525,-1.62672708026858,8.73866951023317E-17));
#11621=CARTESIAN_POINT('Ctrl Pts',(11.7298546566854,1.62699099289774,-0.00505567716946009));
#11622=CARTESIAN_POINT('Ctrl Pts',(11.719037455812,1.61616547398006,0.202324775346606));
#11623=CARTESIAN_POINT('Ctrl Pts',(11.7082205217827,1.60534015781013,0.409705250660816));
#11624=CARTESIAN_POINT('Ctrl Pts',(11.6974038588243,1.59451504727786,0.617085749108931));
#11625=CARTESIAN_POINT('Ctrl Pts',(11.8133862946664,1.61860913476435,-0.00111531114554236));
#11626=CARTESIAN_POINT('Ctrl Pts',(11.8025579038448,1.6077699189899,0.206263846261978));
#11627=CARTESIAN_POINT('Ctrl Pts',(11.7917299466398,1.59693199028804,0.41364309356145));
#11628=CARTESIAN_POINT('Ctrl Pts',(11.7809019683719,1.58609304882157,0.621022283493159));
#11629=CARTESIAN_POINT('Ctrl Pts',(11.9519653779615,1.53884931758497,0.00198566945999789));
#11630=CARTESIAN_POINT('Ctrl Pts',(11.9411087765487,1.52800449744246,0.209363119024413));
#11631=CARTESIAN_POINT('Ctrl Pts',(11.9302521502216,1.51715965702667,0.416740564833343));
#11632=CARTESIAN_POINT('Ctrl Pts',(11.9193956662674,1.50631506689811,0.624118030142866));
#11633=CARTESIAN_POINT('Ctrl Pts',(12.0001655389052,1.39184242582033,-0.00315867047762133));
#11634=CARTESIAN_POINT('Ctrl Pts',(11.9892972278067,1.38101476165208,0.204219175612729));
#11635=CARTESIAN_POINT('Ctrl Pts',(11.9784292129672,1.37018709651964,0.41159703650799));
#11636=CARTESIAN_POINT('Ctrl Pts',(11.9675608998875,1.35935984444403,0.618974903273729));
#11637=CARTESIAN_POINT('Ctrl Pts',(12.0003371960637,1.32889516399154,-0.00643408418199817));
#11638=CARTESIAN_POINT('Ctrl Pts',(11.9894689610601,1.31807475269516,0.200944193475792));
#11639=CARTESIAN_POINT('Ctrl Pts',(11.9786007253947,1.3072545841082,0.408322483762789));
#11640=CARTESIAN_POINT('Ctrl Pts',(11.9677324890572,1.2964346619681,0.615700786872884));
#11641=CARTESIAN_POINT('Ctrl Pts',(11.7295909468525,1.62672708026857,-8.50014503228635E-17));
#11642=CARTESIAN_POINT('Ctrl Pts',(11.7188616535763,1.61598953550924,0.205695227161956));
#11643=CARTESIAN_POINT('Ctrl Pts',(11.7081326228587,1.605252190239,0.411390476755719));
#11644=CARTESIAN_POINT('Ctrl Pts',(11.6974038588243,1.59451504727786,0.617085749108931));
#11645=CARTESIAN_POINT('Ctrl Pts',(11.9677324890572,1.2964346619681,0.615700786872884));
#11646=CARTESIAN_POINT('Ctrl Pts',(11.978488326693,1.30714268506935,0.410467178751997));
#11647=CARTESIAN_POINT('Ctrl Pts',(11.9892441636707,1.31785094954633,0.205233583190349));
#11648=CARTESIAN_POINT('Ctrl Pts',(12.,1.32855945177638,-2.38524477946811E-17));
#11649=CARTESIAN_POINT('Ctrl Pts',(0.3318563713692,1.12115139781563,0.9));
#11650=CARTESIAN_POINT('Ctrl Pts',(1.92849230856897,1.42598364489954,0.9));
#11651=CARTESIAN_POINT('Ctrl Pts',(5.71993880054687,1.76935652211139,0.9));
#11652=CARTESIAN_POINT('Ctrl Pts',(9.51130499016288,1.50815471522196,0.9));
#11653=CARTESIAN_POINT('Ctrl Pts',(11.6681436286308,1.2964346619681,0.9));
#11654=CARTESIAN_POINT('Ctrl Pts',(0.315675209020018,1.2059043252356,0.9));
#11655=CARTESIAN_POINT('Ctrl Pts',(1.91774960754439,1.51208293277137,0.900011072182198));
#11656=CARTESIAN_POINT('Ctrl Pts',(5.72069615836457,1.85663493780214,0.899990666655967));
#11657=CARTESIAN_POINT('Ctrl Pts',(9.5180705084307,1.59456947801794,0.900005849269565));
#11658=CARTESIAN_POINT('Ctrl Pts',(11.6765943959699,1.38252448313292,0.9));
#11659=CARTESIAN_POINT('Ctrl Pts',(0.287623587302861,1.35283178372728,0.83061654407248));
#11660=CARTESIAN_POINT('Ctrl Pts',(1.89907070881462,1.6612970673762,0.830110312711064));
#11661=CARTESIAN_POINT('Ctrl Pts',(5.72203120258494,2.00791989451774,0.829536565111056));
#11662=CARTESIAN_POINT('Ctrl Pts',(9.52981562096212,1.74434245945332,0.829975639897288));
#11663=CARTESIAN_POINT('Ctrl Pts',(11.6912432102654,1.53175516862908,0.830242007927395));
#11664=CARTESIAN_POINT('Ctrl Pts',(0.276437927844243,1.41141950219787,0.682830994206899));
#11665=CARTESIAN_POINT('Ctrl Pts',(1.89175654834445,1.7202459032803,0.681514651829601));
#11666=CARTESIAN_POINT('Ctrl Pts',(5.72254254462207,2.06699613896002,0.680031275065471));
#11667=CARTESIAN_POINT('Ctrl Pts',(9.53442784766217,1.80334383841306,0.681166806353567));
#11668=CARTESIAN_POINT('Ctrl Pts',(11.6970428895979,1.59083777456472,0.681858145263204));
#11669=CARTESIAN_POINT('Ctrl Pts',(0.275700153393682,1.4152837823473,0.618237860411764));
#11670=CARTESIAN_POINT('Ctrl Pts',(1.89131690864814,1.72383635907408,0.616681840548257));
#11671=CARTESIAN_POINT('Ctrl Pts',(5.72257555688819,2.07025489722917,0.614922376024419));
#11672=CARTESIAN_POINT('Ctrl Pts',(9.53470357301702,1.80685728936816,0.616269329673511));
#11673=CARTESIAN_POINT('Ctrl Pts',(11.6974038588243,1.59451504727786,0.617085749108931));
#11674=CARTESIAN_POINT('Ctrl Pts',(11.6974038588243,1.59451504727786,0.617085749108931));
#11675=CARTESIAN_POINT('Ctrl Pts',(9.53470357301702,1.80685728936816,0.616269329673511));
#11676=CARTESIAN_POINT('Ctrl Pts',(5.72257555688819,2.07025489722917,0.614922376024419));
#11677=CARTESIAN_POINT('Ctrl Pts',(1.89131690864814,1.72383635907408,0.616681840548257));
#11678=CARTESIAN_POINT('Ctrl Pts',(0.275700153393682,1.4152837823473,0.618237860411764));
#11679=CARTESIAN_POINT('Ctrl Pts',(0.3318563713692,1.12115139781563,0.9));
#11680=CARTESIAN_POINT('Ctrl Pts',(1.92849230856897,1.42598364489954,0.9));
#11681=CARTESIAN_POINT('Ctrl Pts',(5.71993880054687,1.76935652211139,0.9));
#11682=CARTESIAN_POINT('Ctrl Pts',(9.51130499016288,1.50815471522196,0.9));
#11683=CARTESIAN_POINT('Ctrl Pts',(11.6681436286308,1.2964346619681,0.9));
#11684=CARTESIAN_POINT('Ctrl Pts',(-0.000343174493958709,1.15350944952984,
-0.00654815942696785));
#11685=CARTESIAN_POINT('Ctrl Pts',(0.0105270529019337,1.14272303380391,
0.200868135340743));
#11686=CARTESIAN_POINT('Ctrl Pts',(0.0213972813757523,1.13193701467556,
0.408284450676511));
#11687=CARTESIAN_POINT('Ctrl Pts',(0.0322675109428289,1.12115139781563,
0.615700786872884));
#11688=CARTESIAN_POINT('Ctrl Pts',(-0.000129060241737355,1.23228777111366,
-0.0024626161135415));
#11689=CARTESIAN_POINT('Ctrl Pts',(0.0107416412387167,1.22148297235423,
0.204952596860618));
#11690=CARTESIAN_POINT('Ctrl Pts',(0.0216107531875107,1.21067920461451,
0.412367946918899));
#11691=CARTESIAN_POINT('Ctrl Pts',(0.0324814606290031,1.19987501734845,
0.61978319007907));
#11692=CARTESIAN_POINT('Ctrl Pts',(0.0574602827844584,1.36931747586956,
0.00164530659801973));
#11693=CARTESIAN_POINT('Ctrl Pts',(0.0683025556324749,1.35848226928888,
0.209060253413207));
#11694=CARTESIAN_POINT('Ctrl Pts',(0.079145272670006,1.34764679267913,0.416475160658282));
#11695=CARTESIAN_POINT('Ctrl Pts',(0.0899872847341513,1.33681188280878,
0.62389013300849));
#11696=CARTESIAN_POINT('Ctrl Pts',(0.185325846363896,1.43651931939441,-0.00156109881554352));
#11697=CARTESIAN_POINT('Ctrl Pts',(0.196119220517603,1.4256988926218,0.205857093047737));
#11698=CARTESIAN_POINT('Ctrl Pts',(0.20691256009293,1.41487906031557,0.413275315721495));
#11699=CARTESIAN_POINT('Ctrl Pts',(0.217705180746507,1.40405902353128,0.620693562444772));
#11700=CARTESIAN_POINT('Ctrl Pts',(0.243371723604776,1.44769625339383,-0.00402191236404));
#11701=CARTESIAN_POINT('Ctrl Pts',(0.254148334883323,1.43689183478419,0.203397976373256));
#11702=CARTESIAN_POINT('Ctrl Pts',(0.264924480472538,1.42608767680315,0.410817900476086));
#11703=CARTESIAN_POINT('Ctrl Pts',(0.275700153393682,1.4152837823473,0.618237860411764));
#11704=CARTESIAN_POINT('Ctrl Pts',(-1.23734572934908E-17,1.15316892111333,
-8.67361737988404E-19));
#11705=CARTESIAN_POINT('Ctrl Pts',(0.0107558359204753,1.14249602316336,
0.205233575389367));
#11706=CARTESIAN_POINT('Ctrl Pts',(0.0215116728964674,1.13182351356624,
0.410467170919192));
#11707=CARTESIAN_POINT('Ctrl Pts',(0.0322675109428289,1.12115139781563,
0.615700786872884));
#11708=CARTESIAN_POINT('Ctrl Pts',(0.275700153393682,1.4152837823473,0.618237860411764));
#11709=CARTESIAN_POINT('Ctrl Pts',(0.264994127943615,1.42601784692504,0.412158538389472));
#11710=CARTESIAN_POINT('Ctrl Pts',(0.254287635915814,1.43675217163244,0.206079251738322));
#11711=CARTESIAN_POINT('Ctrl Pts',(0.243580684154575,1.44748675362873,-1.9298798670242E-17));
#11712=CARTESIAN_POINT('Ctrl Pts',(11.7295909468525,-1.62672708026858,0.));
#11713=CARTESIAN_POINT('Ctrl Pts',(11.7192775324813,-1.61592692249094,0.206079286804135));
#11714=CARTESIAN_POINT('Ctrl Pts',(11.70896411811,-1.6051267647133,0.41215857360827));
#11715=CARTESIAN_POINT('Ctrl Pts',(11.6986507037388,-1.59432660693566,0.618237860412405));
#11716=CARTESIAN_POINT('Ctrl Pts',(7.90092085928651,-2.00057770191527,0.));
#11717=CARTESIAN_POINT('Ctrl Pts',(7.89749915175266,-1.98977754413763,0.206079286804135));
#11718=CARTESIAN_POINT('Ctrl Pts',(7.89407744421881,-1.97897738636,0.41215857360827));
#11719=CARTESIAN_POINT('Ctrl Pts',(7.89065573668496,-1.96817722858236,0.618237860412405));
#11720=CARTESIAN_POINT('Ctrl Pts',(4.07225077172054,-2.17467835246083,0.));
#11721=CARTESIAN_POINT('Ctrl Pts',(4.07572077102407,-2.16387819468319,0.206079286804135));
#11722=CARTESIAN_POINT('Ctrl Pts',(4.07919077032759,-2.15307803690555,0.41215857360827));
#11723=CARTESIAN_POINT('Ctrl Pts',(4.08266076963111,-2.14227787912792,0.618237860412405));
#11724=CARTESIAN_POINT('Ctrl Pts',(0.243580684154574,-1.44748675362873,
0.));
#11725=CARTESIAN_POINT('Ctrl Pts',(0.253942390295469,-1.43668659585109,
0.206079286804135));
#11726=CARTESIAN_POINT('Ctrl Pts',(0.264304096436365,-1.42588643807345,
0.41215857360827));
#11727=CARTESIAN_POINT('Ctrl Pts',(0.27466580257726,-1.41508628029581,0.618237860412405));
#11728=CARTESIAN_POINT('Origin',(0.,-1.4,0.));
#11729=CARTESIAN_POINT('Origin',(6.08012166120517,1.06803409199199E-16,
0.9));
#11730=CARTESIAN_POINT('Ctrl Pts',(0.243580684154574,1.44748675362873,0.));
#11731=CARTESIAN_POINT('Ctrl Pts',(0.253942390295469,1.43668659585109,0.206079286804135));
#11732=CARTESIAN_POINT('Ctrl Pts',(0.264304096436365,1.42588643807345,0.41215857360827));
#11733=CARTESIAN_POINT('Ctrl Pts',(0.27466580257726,1.41508628029581,0.618237860412405));
#11734=CARTESIAN_POINT('Ctrl Pts',(4.07225077172054,2.17467835246083,0.));
#11735=CARTESIAN_POINT('Ctrl Pts',(4.07572077102407,2.16387819468319,0.206079286804135));
#11736=CARTESIAN_POINT('Ctrl Pts',(4.07919077032759,2.15307803690555,0.41215857360827));
#11737=CARTESIAN_POINT('Ctrl Pts',(4.08266076963111,2.14227787912792,0.618237860412405));
#11738=CARTESIAN_POINT('Ctrl Pts',(7.90092085928651,2.00057770191527,0.));
#11739=CARTESIAN_POINT('Ctrl Pts',(7.89749915175266,1.98977754413763,0.206079286804135));
#11740=CARTESIAN_POINT('Ctrl Pts',(7.89407744421881,1.97897738636,0.41215857360827));
#11741=CARTESIAN_POINT('Ctrl Pts',(7.89065573668496,1.96817722858236,0.618237860412405));
#11742=CARTESIAN_POINT('Ctrl Pts',(11.7295909468525,1.62672708026858,0.));
#11743=CARTESIAN_POINT('Ctrl Pts',(11.7192775324813,1.61592692249094,0.206079286804135));
#11744=CARTESIAN_POINT('Ctrl Pts',(11.70896411811,1.6051267647133,0.41215857360827));
#11745=CARTESIAN_POINT('Ctrl Pts',(11.6986507037388,1.59432660693566,0.618237860412405));
#11746=CARTESIAN_POINT('Origin',(12.,1.6,0.));
#19452=UNCERTAINTY_MEASURE_WITH_UNIT(LENGTH_MEASURE(0.001),#19472,
'DISTANCE_ACCURACY_VALUE',
'Maximum model space distance between geometric entities at asserted c
onnectivities');
#19458=UNCERTAINTY_MEASURE_WITH_UNIT(LENGTH_MEASURE(0.001),#19472,
'DISTANCE_ACCURACY_VALUE',
'Maximum model space distance between geometric entities at asserted c
onnectivities');
#19465=(
GEOMETRIC_REPRESENTATION_CONTEXT(3)
GLOBAL_UNCERTAINTY_ASSIGNED_CONTEXT((#19452))
GLOBAL_UNIT_ASSIGNED_CONTEXT((#19472,#19474,#19475))
REPRESENTATION_CONTEXT('','3D')
);
#19471=(
GEOMETRIC_REPRESENTATION_CONTEXT(3)
GLOBAL_UNCERTAINTY_ASSIGNED_CONTEXT((#19458))
GLOBAL_UNIT_ASSIGNED_CONTEXT((#19472,#19474,#19475))
REPRESENTATION_CONTEXT('','3D')
);
#19472=(
LENGTH_UNIT()
NAMED_UNIT(*)
SI_UNIT(.CENTI.,.METRE.)
);
#19474=(
NAMED_UNIT(*)
PLANE_ANGLE_UNIT()
SI_UNIT($,.RADIAN.)
);
#19475=(
NAMED_UNIT(*)
SI_UNIT($,.STERADIAN.)
SOLID_ANGLE_UNIT()
);
#19482=SHAPE_DEFINITION_REPRESENTATION(#19494,#19522);
#19494=PRODUCT_DEFINITION_SHAPE('',$,#19535);
#19522=SHAPE_REPRESENTATION('',(#7423),#19465);
#19528=PRODUCT_DEFINITION_CONTEXT('part definition',#19566,'design');
#19535=PRODUCT_DEFINITION('2026-11-10-01-30-02-385',
'Upper structural shell',#19547,#19528);
#19547=PRODUCT_DEFINITION_FORMATION('',$,#19574);
#19566=APPLICATION_CONTEXT(
'Core Data for Automotive Mechanical Design Process');
#19567=PRODUCT_CONTEXT('part definition',#19566,'mechanical');
#19574=PRODUCT('2026-11-10-01-30-02-385','Upper structural shell',$,(#19567));
#19584=PRESENTATION_STYLE_ASSIGNMENT((#19592));
#19592=SURFACE_STYLE_USAGE(.BOTH.,#19600);
#19600=SURFACE_SIDE_STYLE('',(#19608));
#19608=SURFACE_STYLE_FILL_AREA(#19616);
#19616=FILL_AREA_STYLE('Structural dark blue',(#19624));
#19624=FILL_AREA_STYLE_COLOUR('Structural dark blue',#19632);
#19632=COLOUR_RGB('Structural dark blue',0.0901960784313725,0.270588235294118,
0.513725490196078);
ENDSEC;
END-ISO-10303-21;
